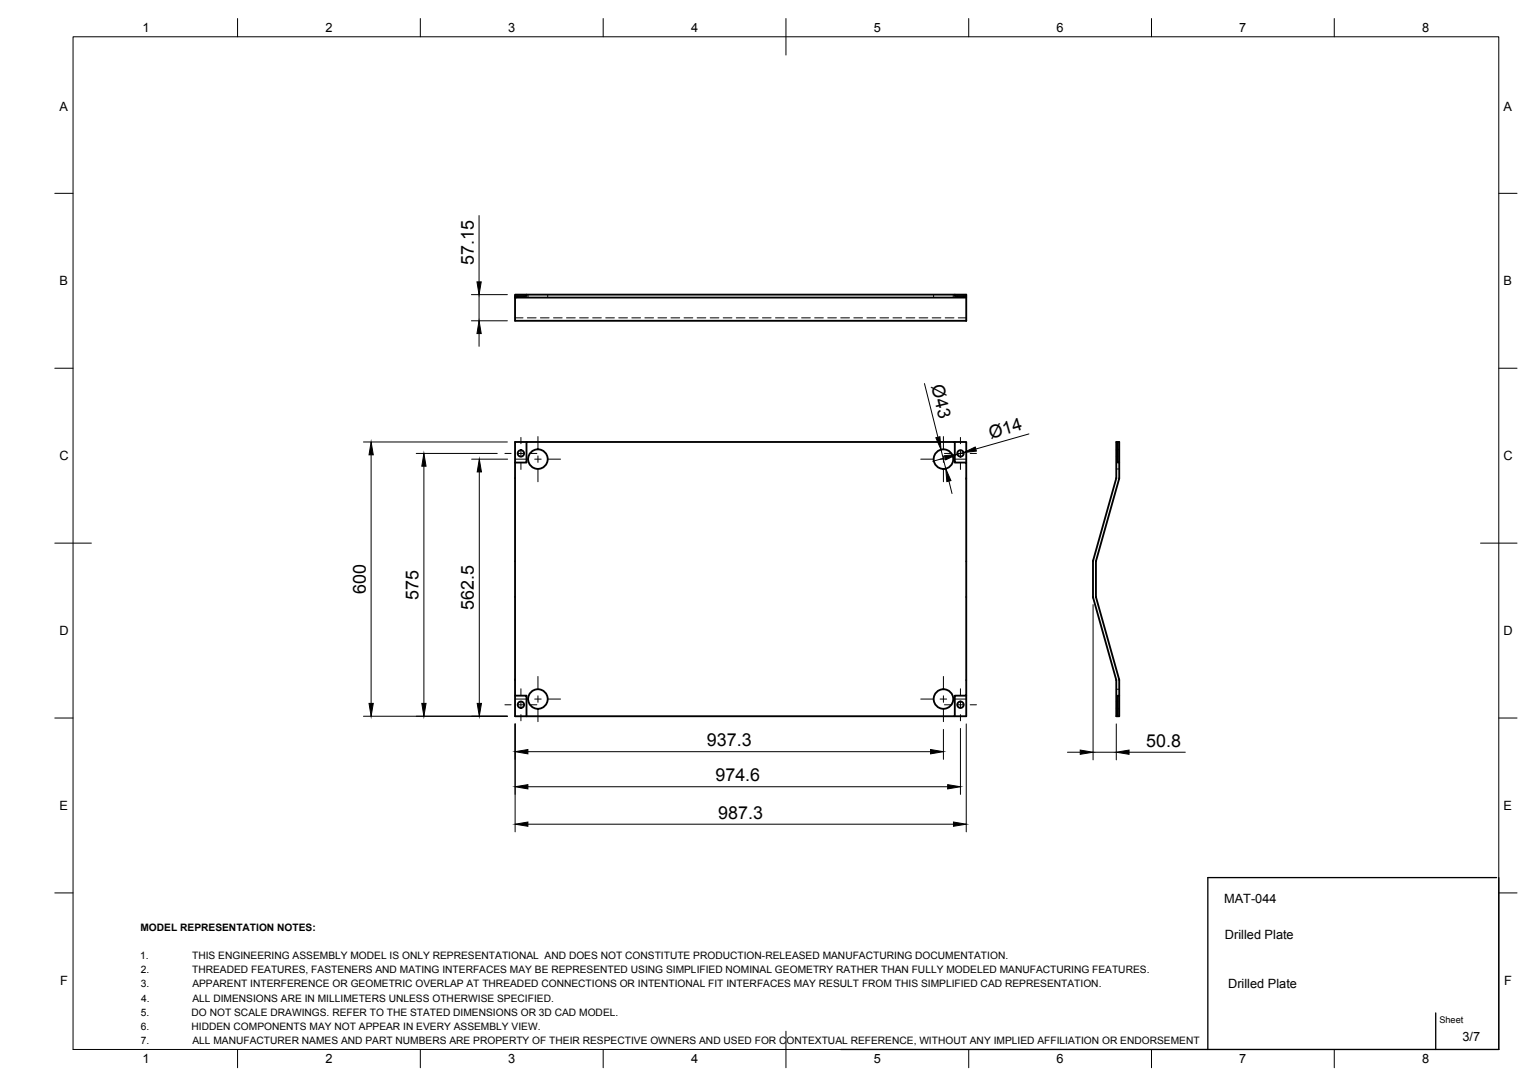
ISO-10303-21;
HEADER;
/* Generated by software containing ST-Developer
 * from STEP Tools, Inc. (www.steptools.com) 
 */

FILE_DESCRIPTION(
/* description */ ('STEP AP214'),
/* implementation_level */ '2;1');

FILE_NAME(
/* name */ 'Drilled Plate.step',
/* time_stamp */ '2026-11-14T22:20:24-08:00',
/* author */ (''),
/* organization */ (''),
/* preprocessor_version */ 'ST-DEVELOPER v20.2',
/* originating_system */ 'Autodesk Translation Framework v15.17.0.0',
/* authorisation */ '');

FILE_SCHEMA (('AUTOMOTIVE_DESIGN { 1 0 10303 214 3 1 1 }'));
ENDSEC;

DATA;
#10=MECHANICAL_DESIGN_GEOMETRIC_PRESENTATION_REPRESENTATION('',(#82),#2794);
#72=SHAPE_REPRESENTATION_RELATIONSHIP('SRR','None',#2827,#77);
#77=ADVANCED_BREP_SHAPE_REPRESENTATION('',(#87),#2789);
#82=STYLED_ITEM('',(#2861),#87);
#87=MANIFOLD_SOLID_BREP('Body1',#1641);
#92=FACE_BOUND('',#286,.T.);
#93=FACE_BOUND('',#287,.T.);
#94=FACE_BOUND('',#288,.T.);
#95=FACE_BOUND('',#289,.T.);
#96=FACE_BOUND('',#291,.T.);
#97=FACE_BOUND('',#292,.T.);
#98=FACE_BOUND('',#293,.T.);
#99=FACE_BOUND('',#294,.T.);
#100=FACE_BOUND('',#296,.T.);
#101=FACE_BOUND('',#297,.T.);
#102=FACE_BOUND('',#299,.T.);
#103=FACE_BOUND('',#300,.T.);
#104=FACE_BOUND('',#338,.T.);
#105=FACE_BOUND('',#342,.T.);
#106=FACE_BOUND('',#346,.T.);
#107=FACE_BOUND('',#350,.T.);
#116=PLANE('',#1728);
#117=PLANE('',#1729);
#118=PLANE('',#1730);
#119=PLANE('',#1731);
#120=PLANE('',#1732);
#121=PLANE('',#1733);
#122=PLANE('',#1734);
#123=PLANE('',#1735);
#124=PLANE('',#1736);
#125=PLANE('',#1739);
#126=PLANE('',#1740);
#127=PLANE('',#1743);
#128=PLANE('',#1746);
#129=PLANE('',#1747);
#130=PLANE('',#1750);
#131=PLANE('',#1751);
#132=PLANE('',#1754);
#133=PLANE('',#1755);
#134=PLANE('',#1758);
#135=PLANE('',#1759);
#136=PLANE('',#1762);
#137=PLANE('',#1765);
#138=PLANE('',#1767);
#139=PLANE('',#1769);
#140=PLANE('',#1771);
#141=PLANE('',#1774);
#142=PLANE('',#1776);
#143=PLANE('',#1778);
#144=PLANE('',#1780);
#145=PLANE('',#1781);
#146=PLANE('',#1782);
#147=PLANE('',#1783);
#148=PLANE('',#1784);
#149=PLANE('',#1785);
#150=PLANE('',#1786);
#151=PLANE('',#1787);
#152=PLANE('',#1788);
#153=PLANE('',#1789);
#154=PLANE('',#1790);
#155=PLANE('',#1791);
#156=PLANE('',#1792);
#157=PLANE('',#1793);
#186=FACE_OUTER_BOUND('',#277,.T.);
#187=FACE_OUTER_BOUND('',#278,.T.);
#188=FACE_OUTER_BOUND('',#279,.T.);
#189=FACE_OUTER_BOUND('',#280,.T.);
#190=FACE_OUTER_BOUND('',#281,.T.);
#191=FACE_OUTER_BOUND('',#282,.T.);
#192=FACE_OUTER_BOUND('',#283,.T.);
#193=FACE_OUTER_BOUND('',#284,.T.);
#194=FACE_OUTER_BOUND('',#285,.T.);
#195=FACE_OUTER_BOUND('',#290,.T.);
#196=FACE_OUTER_BOUND('',#295,.T.);
#197=FACE_OUTER_BOUND('',#298,.T.);
#198=FACE_OUTER_BOUND('',#301,.T.);
#199=FACE_OUTER_BOUND('',#302,.T.);
#200=FACE_OUTER_BOUND('',#303,.T.);
#201=FACE_OUTER_BOUND('',#304,.T.);
#202=FACE_OUTER_BOUND('',#305,.T.);
#203=FACE_OUTER_BOUND('',#306,.T.);
#204=FACE_OUTER_BOUND('',#307,.T.);
#205=FACE_OUTER_BOUND('',#308,.T.);
#206=FACE_OUTER_BOUND('',#309,.T.);
#207=FACE_OUTER_BOUND('',#310,.T.);
#208=FACE_OUTER_BOUND('',#311,.T.);
#209=FACE_OUTER_BOUND('',#312,.T.);
#210=FACE_OUTER_BOUND('',#313,.T.);
#211=FACE_OUTER_BOUND('',#314,.T.);
#212=FACE_OUTER_BOUND('',#315,.T.);
#213=FACE_OUTER_BOUND('',#316,.T.);
#214=FACE_OUTER_BOUND('',#317,.T.);
#215=FACE_OUTER_BOUND('',#318,.T.);
#216=FACE_OUTER_BOUND('',#319,.T.);
#217=FACE_OUTER_BOUND('',#320,.T.);
#218=FACE_OUTER_BOUND('',#321,.T.);
#219=FACE_OUTER_BOUND('',#322,.T.);
#220=FACE_OUTER_BOUND('',#323,.T.);
#221=FACE_OUTER_BOUND('',#324,.T.);
#222=FACE_OUTER_BOUND('',#325,.T.);
#223=FACE_OUTER_BOUND('',#326,.T.);
#224=FACE_OUTER_BOUND('',#327,.T.);
#225=FACE_OUTER_BOUND('',#328,.T.);
#226=FACE_OUTER_BOUND('',#329,.T.);
#227=FACE_OUTER_BOUND('',#330,.T.);
#228=FACE_OUTER_BOUND('',#331,.T.);
#229=FACE_OUTER_BOUND('',#332,.T.);
#230=FACE_OUTER_BOUND('',#333,.T.);
#231=FACE_OUTER_BOUND('',#334,.T.);
#232=FACE_OUTER_BOUND('',#335,.T.);
#233=FACE_OUTER_BOUND('',#336,.T.);
#234=FACE_OUTER_BOUND('',#337,.T.);
#235=FACE_OUTER_BOUND('',#339,.T.);
#236=FACE_OUTER_BOUND('',#340,.T.);
#237=FACE_OUTER_BOUND('',#341,.T.);
#238=FACE_OUTER_BOUND('',#343,.T.);
#239=FACE_OUTER_BOUND('',#344,.T.);
#240=FACE_OUTER_BOUND('',#345,.T.);
#241=FACE_OUTER_BOUND('',#347,.T.);
#242=FACE_OUTER_BOUND('',#348,.T.);
#243=FACE_OUTER_BOUND('',#349,.T.);
#277=EDGE_LOOP('',(#1110,#1111,#1112,#1113));
#278=EDGE_LOOP('',(#1114,#1115,#1116,#1117));
#279=EDGE_LOOP('',(#1118,#1119,#1120,#1121));
#280=EDGE_LOOP('',(#1122,#1123,#1124,#1125));
#281=EDGE_LOOP('',(#1126,#1127,#1128,#1129));
#282=EDGE_LOOP('',(#1130,#1131,#1132,#1133));
#283=EDGE_LOOP('',(#1134,#1135,#1136,#1137));
#284=EDGE_LOOP('',(#1138,#1139,#1140,#1141));
#285=EDGE_LOOP('',(#1142,#1143,#1144,#1145));
#286=EDGE_LOOP('',(#1146));
#287=EDGE_LOOP('',(#1147));
#288=EDGE_LOOP('',(#1148));
#289=EDGE_LOOP('',(#1149));
#290=EDGE_LOOP('',(#1150,#1151,#1152,#1153));
#291=EDGE_LOOP('',(#1154));
#292=EDGE_LOOP('',(#1155));
#293=EDGE_LOOP('',(#1156));
#294=EDGE_LOOP('',(#1157));
#295=EDGE_LOOP('',(#1158,#1159,#1160,#1161,#1162,#1163,#1164,#1165));
#296=EDGE_LOOP('',(#1166));
#297=EDGE_LOOP('',(#1167));
#298=EDGE_LOOP('',(#1168,#1169,#1170,#1171,#1172,#1173,#1174,#1175));
#299=EDGE_LOOP('',(#1176));
#300=EDGE_LOOP('',(#1177));
#301=EDGE_LOOP('',(#1178,#1179,#1180,#1181,#1182,#1183));
#302=EDGE_LOOP('',(#1184,#1185,#1186,#1187,#1188,#1189));
#303=EDGE_LOOP('',(#1190,#1191,#1192,#1193,#1194,#1195,#1196,#1197));
#304=EDGE_LOOP('',(#1198,#1199,#1200,#1201,#1202,#1203,#1204,#1205));
#305=EDGE_LOOP('',(#1206,#1207,#1208,#1209));
#306=EDGE_LOOP('',(#1210,#1211,#1212,#1213));
#307=EDGE_LOOP('',(#1214,#1215,#1216,#1217));
#308=EDGE_LOOP('',(#1218,#1219,#1220,#1221));
#309=EDGE_LOOP('',(#1222,#1223,#1224,#1225));
#310=EDGE_LOOP('',(#1226,#1227,#1228,#1229));
#311=EDGE_LOOP('',(#1230,#1231,#1232,#1233));
#312=EDGE_LOOP('',(#1234,#1235,#1236,#1237));
#313=EDGE_LOOP('',(#1238,#1239,#1240,#1241));
#314=EDGE_LOOP('',(#1242,#1243,#1244,#1245));
#315=EDGE_LOOP('',(#1246,#1247,#1248,#1249));
#316=EDGE_LOOP('',(#1250,#1251,#1252,#1253));
#317=EDGE_LOOP('',(#1254,#1255,#1256,#1257));
#318=EDGE_LOOP('',(#1258,#1259,#1260,#1261));
#319=EDGE_LOOP('',(#1262,#1263,#1264,#1265));
#320=EDGE_LOOP('',(#1266,#1267,#1268,#1269));
#321=EDGE_LOOP('',(#1270,#1271,#1272,#1273));
#322=EDGE_LOOP('',(#1274,#1275,#1276,#1277));
#323=EDGE_LOOP('',(#1278,#1279,#1280,#1281));
#324=EDGE_LOOP('',(#1282,#1283,#1284,#1285));
#325=EDGE_LOOP('',(#1286,#1287,#1288,#1289));
#326=EDGE_LOOP('',(#1290,#1291,#1292,#1293));
#327=EDGE_LOOP('',(#1294,#1295,#1296,#1297));
#328=EDGE_LOOP('',(#1298,#1299,#1300,#1301));
#329=EDGE_LOOP('',(#1302,#1303,#1304,#1305));
#330=EDGE_LOOP('',(#1306,#1307,#1308,#1309));
#331=EDGE_LOOP('',(#1310,#1311,#1312,#1313));
#332=EDGE_LOOP('',(#1314,#1315,#1316,#1317));
#333=EDGE_LOOP('',(#1318,#1319,#1320,#1321,#1322,#1323));
#334=EDGE_LOOP('',(#1324,#1325,#1326,#1327,#1328,#1329));
#335=EDGE_LOOP('',(#1330,#1331,#1332,#1333));
#336=EDGE_LOOP('',(#1334,#1335,#1336,#1337));
#337=EDGE_LOOP('',(#1338,#1339,#1340,#1341));
#338=EDGE_LOOP('',(#1342));
#339=EDGE_LOOP('',(#1343,#1344,#1345,#1346));
#340=EDGE_LOOP('',(#1347,#1348,#1349,#1350));
#341=EDGE_LOOP('',(#1351,#1352,#1353,#1354));
#342=EDGE_LOOP('',(#1355));
#343=EDGE_LOOP('',(#1356,#1357,#1358,#1359));
#344=EDGE_LOOP('',(#1360,#1361,#1362,#1363));
#345=EDGE_LOOP('',(#1364,#1365,#1366,#1367));
#346=EDGE_LOOP('',(#1368));
#347=EDGE_LOOP('',(#1369,#1370,#1371,#1372));
#348=EDGE_LOOP('',(#1373,#1374,#1375,#1376));
#349=EDGE_LOOP('',(#1377,#1378,#1379,#1380));
#350=EDGE_LOOP('',(#1381));
#392=LINE('',#2336,#561);
#393=LINE('',#2342,#562);
#394=LINE('',#2348,#563);
#395=LINE('',#2354,#564);
#396=LINE('',#2360,#565);
#397=LINE('',#2366,#566);
#398=LINE('',#2372,#567);
#399=LINE('',#2378,#568);
#400=LINE('',#2383,#569);
#401=LINE('',#2385,#570);
#402=LINE('',#2387,#571);
#403=LINE('',#2388,#572);
#404=LINE('',#2392,#573);
#405=LINE('',#2394,#574);
#406=LINE('',#2396,#575);
#407=LINE('',#2397,#576);
#408=LINE('',#2401,#577);
#409=LINE('',#2403,#578);
#410=LINE('',#2405,#579);
#411=LINE('',#2407,#580);
#412=LINE('',#2409,#581);
#413=LINE('',#2411,#582);
#414=LINE('',#2413,#583);
#415=LINE('',#2414,#584);
#416=LINE('',#2418,#585);
#417=LINE('',#2420,#586);
#418=LINE('',#2422,#587);
#419=LINE('',#2424,#588);
#420=LINE('',#2426,#589);
#421=LINE('',#2428,#590);
#422=LINE('',#2430,#591);
#423=LINE('',#2431,#592);
#424=LINE('',#2435,#593);
#425=LINE('',#2436,#594);
#426=LINE('',#2437,#595);
#427=LINE('',#2438,#596);
#428=LINE('',#2442,#597);
#429=LINE('',#2443,#598);
#430=LINE('',#2444,#599);
#431=LINE('',#2445,#600);
#432=LINE('',#2448,#601);
#433=LINE('',#2449,#602);
#434=LINE('',#2451,#603);
#435=LINE('',#2453,#604);
#436=LINE('',#2454,#605);
#437=LINE('',#2458,#606);
#438=LINE('',#2459,#607);
#439=LINE('',#2461,#608);
#440=LINE('',#2462,#609);
#441=LINE('',#2463,#610);
#442=LINE('',#2467,#611);
#443=LINE('',#2469,#612);
#444=LINE('',#2473,#613);
#445=LINE('',#2475,#614);
#446=LINE('',#2476,#615);
#447=LINE('',#2481,#616);
#448=LINE('',#2486,#617);
#449=LINE('',#2491,#618);
#450=LINE('',#2493,#619);
#451=LINE('',#2494,#620);
#452=LINE('',#2498,#621);
#453=LINE('',#2502,#622);
#454=LINE('',#2505,#623);
#455=LINE('',#2506,#624);
#456=LINE('',#2510,#625);
#457=LINE('',#2515,#626);
#458=LINE('',#2517,#627);
#459=LINE('',#2518,#628);
#460=LINE('',#2522,#629);
#461=LINE('',#2526,#630);
#462=LINE('',#2529,#631);
#463=LINE('',#2530,#632);
#464=LINE('',#2537,#633);
#465=LINE('',#2539,#634);
#466=LINE('',#2542,#635);
#467=LINE('',#2543,#636);
#468=LINE('',#2545,#637);
#469=LINE('',#2547,#638);
#470=LINE('',#2549,#639);
#471=LINE('',#2551,#640);
#472=LINE('',#2553,#641);
#473=LINE('',#2555,#642);
#474=LINE('',#2558,#643);
#475=LINE('',#2560,#644);
#476=LINE('',#2562,#645);
#477=LINE('',#2564,#646);
#478=LINE('',#2566,#647);
#479=LINE('',#2568,#648);
#480=LINE('',#2572,#649);
#481=LINE('',#2573,#650);
#482=LINE('',#2576,#651);
#483=LINE('',#2577,#652);
#484=LINE('',#2580,#653);
#485=LINE('',#2581,#654);
#486=LINE('',#2583,#655);
#487=LINE('',#2587,#656);
#488=LINE('',#2588,#657);
#489=LINE('',#2590,#658);
#490=LINE('',#2594,#659);
#491=LINE('',#2595,#660);
#492=LINE('',#2597,#661);
#493=LINE('',#2601,#662);
#494=LINE('',#2602,#663);
#495=LINE('',#2604,#664);
#561=VECTOR('',#1863,6.99999999999993);
#562=VECTOR('',#1870,7.00000000000001);
#563=VECTOR('',#1877,6.99999999999996);
#564=VECTOR('',#1884,6.9999999999999);
#565=VECTOR('',#1891,21.5);
#566=VECTOR('',#1898,21.5);
#567=VECTOR('',#1905,21.5);
#568=VECTOR('',#1912,21.5);
#569=VECTOR('',#1917,1000.);
#570=VECTOR('',#1918,1000.);
#571=VECTOR('',#1919,1000.);
#572=VECTOR('',#1920,1000.);
#573=VECTOR('',#1923,1000.);
#574=VECTOR('',#1924,1000.);
#575=VECTOR('',#1925,1000.);
#576=VECTOR('',#1926,1000.);
#577=VECTOR('',#1929,1000.);
#578=VECTOR('',#1930,1000.);
#579=VECTOR('',#1931,1000.);
#580=VECTOR('',#1932,1000.);
#581=VECTOR('',#1933,1000.);
#582=VECTOR('',#1934,1000.);
#583=VECTOR('',#1935,1000.);
#584=VECTOR('',#1936,1000.);
#585=VECTOR('',#1939,1000.);
#586=VECTOR('',#1940,1000.);
#587=VECTOR('',#1941,1000.);
#588=VECTOR('',#1942,1000.);
#589=VECTOR('',#1943,1000.);
#590=VECTOR('',#1944,1000.);
#591=VECTOR('',#1945,1000.);
#592=VECTOR('',#1946,1000.);
#593=VECTOR('',#1949,1000.);
#594=VECTOR('',#1950,1000.);
#595=VECTOR('',#1951,1000.);
#596=VECTOR('',#1952,1000.);
#597=VECTOR('',#1955,1000.);
#598=VECTOR('',#1956,1000.);
#599=VECTOR('',#1957,1000.);
#600=VECTOR('',#1958,1000.);
#601=VECTOR('',#1961,1000.);
#602=VECTOR('',#1962,1000.);
#603=VECTOR('',#1963,1000.);
#604=VECTOR('',#1964,1000.);
#605=VECTOR('',#1965,1000.);
#606=VECTOR('',#1968,1000.);
#607=VECTOR('',#1969,1000.);
#608=VECTOR('',#1970,1000.);
#609=VECTOR('',#1971,1000.);
#610=VECTOR('',#1972,1000.);
#611=VECTOR('',#1975,1000.);
#612=VECTOR('',#1978,1000.);
#613=VECTOR('',#1983,1000.);
#614=VECTOR('',#1984,1000.);
#615=VECTOR('',#1985,1000.);
#616=VECTOR('',#1990,1000.);
#617=VECTOR('',#1995,1000.);
#618=VECTOR('',#2002,1000.);
#619=VECTOR('',#2003,1000.);
#620=VECTOR('',#2004,1000.);
#621=VECTOR('',#2007,1000.);
#622=VECTOR('',#2010,1000.);
#623=VECTOR('',#2015,1000.);
#624=VECTOR('',#2016,1000.);
#625=VECTOR('',#2019,1000.);
#626=VECTOR('',#2026,1000.);
#627=VECTOR('',#2027,1000.);
#628=VECTOR('',#2028,1000.);
#629=VECTOR('',#2031,1000.);
#630=VECTOR('',#2034,1000.);
#631=VECTOR('',#2039,1000.);
#632=VECTOR('',#2040,1000.);
#633=VECTOR('',#2049,1000.);
#634=VECTOR('',#2052,1000.);
#635=VECTOR('',#2057,1000.);
#636=VECTOR('',#2058,1000.);
#637=VECTOR('',#2061,1000.);
#638=VECTOR('',#2064,1000.);
#639=VECTOR('',#2067,1000.);
#640=VECTOR('',#2070,1000.);
#641=VECTOR('',#2073,1000.);
#642=VECTOR('',#2076,1000.);
#643=VECTOR('',#2081,1000.);
#644=VECTOR('',#2084,1000.);
#645=VECTOR('',#2087,1000.);
#646=VECTOR('',#2090,1000.);
#647=VECTOR('',#2093,1000.);
#648=VECTOR('',#2096,1000.);
#649=VECTOR('',#2101,1000.);
#650=VECTOR('',#2102,1000.);
#651=VECTOR('',#2105,1000.);
#652=VECTOR('',#2106,1000.);
#653=VECTOR('',#2109,1000.);
#654=VECTOR('',#2110,1000.);
#655=VECTOR('',#2113,1000.);
#656=VECTOR('',#2118,1000.);
#657=VECTOR('',#2119,1000.);
#658=VECTOR('',#2122,1000.);
#659=VECTOR('',#2127,1000.);
#660=VECTOR('',#2128,1000.);
#661=VECTOR('',#2131,1000.);
#662=VECTOR('',#2136,1000.);
#663=VECTOR('',#2137,1000.);
#664=VECTOR('',#2140,1000.);
#730=CIRCLE('',#1705,6.99999999999992);
#731=CIRCLE('',#1706,6.99999999999992);
#732=CIRCLE('',#1708,7.00000000000001);
#733=CIRCLE('',#1709,7.00000000000001);
#734=CIRCLE('',#1711,6.99999999999996);
#735=CIRCLE('',#1712,6.99999999999996);
#736=CIRCLE('',#1714,6.9999999999999);
#737=CIRCLE('',#1715,6.9999999999999);
#738=CIRCLE('',#1717,21.5);
#739=CIRCLE('',#1718,21.5);
#740=CIRCLE('',#1720,21.5);
#741=CIRCLE('',#1721,21.5);
#742=CIRCLE('',#1723,21.5);
#743=CIRCLE('',#1724,21.5);
#744=CIRCLE('',#1726,21.5);
#745=CIRCLE('',#1727,21.5);
#746=CIRCLE('',#1737,7.35);
#747=CIRCLE('',#1738,1.);
#748=CIRCLE('',#1741,7.35);
#749=CIRCLE('',#1742,1.);
#750=CIRCLE('',#1744,1.);
#751=CIRCLE('',#1745,7.35000000000002);
#752=CIRCLE('',#1748,1.);
#753=CIRCLE('',#1749,7.35000000000002);
#754=CIRCLE('',#1752,1.);
#755=CIRCLE('',#1753,7.35000000000002);
#756=CIRCLE('',#1756,1.);
#757=CIRCLE('',#1757,7.35000000000002);
#758=CIRCLE('',#1760,7.34999999999997);
#759=CIRCLE('',#1761,1.);
#760=CIRCLE('',#1763,7.34999999999997);
#761=CIRCLE('',#1764,1.);
#771=VERTEX_POINT('',#2333);
#772=VERTEX_POINT('',#2335);
#773=VERTEX_POINT('',#2339);
#774=VERTEX_POINT('',#2341);
#775=VERTEX_POINT('',#2345);
#776=VERTEX_POINT('',#2347);
#777=VERTEX_POINT('',#2351);
#778=VERTEX_POINT('',#2353);
#779=VERTEX_POINT('',#2357);
#780=VERTEX_POINT('',#2359);
#781=VERTEX_POINT('',#2363);
#782=VERTEX_POINT('',#2365);
#783=VERTEX_POINT('',#2369);
#784=VERTEX_POINT('',#2371);
#785=VERTEX_POINT('',#2375);
#786=VERTEX_POINT('',#2377);
#787=VERTEX_POINT('',#2381);
#788=VERTEX_POINT('',#2382);
#789=VERTEX_POINT('',#2384);
#790=VERTEX_POINT('',#2386);
#791=VERTEX_POINT('',#2390);
#792=VERTEX_POINT('',#2391);
#793=VERTEX_POINT('',#2393);
#794=VERTEX_POINT('',#2395);
#795=VERTEX_POINT('',#2399);
#796=VERTEX_POINT('',#2400);
#797=VERTEX_POINT('',#2402);
#798=VERTEX_POINT('',#2404);
#799=VERTEX_POINT('',#2406);
#800=VERTEX_POINT('',#2408);
#801=VERTEX_POINT('',#2410);
#802=VERTEX_POINT('',#2412);
#803=VERTEX_POINT('',#2416);
#804=VERTEX_POINT('',#2417);
#805=VERTEX_POINT('',#2419);
#806=VERTEX_POINT('',#2421);
#807=VERTEX_POINT('',#2423);
#808=VERTEX_POINT('',#2425);
#809=VERTEX_POINT('',#2427);
#810=VERTEX_POINT('',#2429);
#811=VERTEX_POINT('',#2433);
#812=VERTEX_POINT('',#2434);
#813=VERTEX_POINT('',#2440);
#814=VERTEX_POINT('',#2441);
#815=VERTEX_POINT('',#2447);
#816=VERTEX_POINT('',#2450);
#817=VERTEX_POINT('',#2452);
#818=VERTEX_POINT('',#2456);
#819=VERTEX_POINT('',#2457);
#820=VERTEX_POINT('',#2460);
#821=VERTEX_POINT('',#2465);
#822=VERTEX_POINT('',#2466);
#823=VERTEX_POINT('',#2472);
#824=VERTEX_POINT('',#2474);
#825=VERTEX_POINT('',#2478);
#826=VERTEX_POINT('',#2480);
#827=VERTEX_POINT('',#2484);
#828=VERTEX_POINT('',#2485);
#829=VERTEX_POINT('',#2490);
#830=VERTEX_POINT('',#2492);
#831=VERTEX_POINT('',#2496);
#832=VERTEX_POINT('',#2497);
#833=VERTEX_POINT('',#2499);
#834=VERTEX_POINT('',#2501);
#835=VERTEX_POINT('',#2508);
#836=VERTEX_POINT('',#2509);
#837=VERTEX_POINT('',#2514);
#838=VERTEX_POINT('',#2516);
#839=VERTEX_POINT('',#2520);
#840=VERTEX_POINT('',#2521);
#841=VERTEX_POINT('',#2523);
#842=VERTEX_POINT('',#2525);
#843=VERTEX_POINT('',#2535);
#844=VERTEX_POINT('',#2536);
#845=VERTEX_POINT('',#2571);
#846=VERTEX_POINT('',#2575);
#847=VERTEX_POINT('',#2579);
#848=VERTEX_POINT('',#2586);
#849=VERTEX_POINT('',#2593);
#850=VERTEX_POINT('',#2600);
#900=EDGE_CURVE('',#771,#771,#730,.T.);
#901=EDGE_CURVE('',#771,#772,#392,.T.);
#902=EDGE_CURVE('',#772,#772,#731,.T.);
#903=EDGE_CURVE('',#773,#773,#732,.T.);
#904=EDGE_CURVE('',#773,#774,#393,.T.);
#905=EDGE_CURVE('',#774,#774,#733,.T.);
#906=EDGE_CURVE('',#775,#775,#734,.T.);
#907=EDGE_CURVE('',#775,#776,#394,.T.);
#908=EDGE_CURVE('',#776,#776,#735,.T.);
#909=EDGE_CURVE('',#777,#777,#736,.T.);
#910=EDGE_CURVE('',#777,#778,#395,.T.);
#911=EDGE_CURVE('',#778,#778,#737,.T.);
#912=EDGE_CURVE('',#779,#779,#738,.T.);
#913=EDGE_CURVE('',#779,#780,#396,.T.);
#914=EDGE_CURVE('',#780,#780,#739,.T.);
#915=EDGE_CURVE('',#781,#781,#740,.T.);
#916=EDGE_CURVE('',#781,#782,#397,.T.);
#917=EDGE_CURVE('',#782,#782,#741,.T.);
#918=EDGE_CURVE('',#783,#783,#742,.T.);
#919=EDGE_CURVE('',#783,#784,#398,.T.);
#920=EDGE_CURVE('',#784,#784,#743,.T.);
#921=EDGE_CURVE('',#785,#785,#744,.T.);
#922=EDGE_CURVE('',#785,#786,#399,.T.);
#923=EDGE_CURVE('',#786,#786,#745,.T.);
#924=EDGE_CURVE('',#787,#788,#400,.T.);
#925=EDGE_CURVE('',#789,#788,#401,.T.);
#926=EDGE_CURVE('',#790,#789,#402,.T.);
#927=EDGE_CURVE('',#790,#787,#403,.T.);
#928=EDGE_CURVE('',#791,#792,#404,.T.);
#929=EDGE_CURVE('',#793,#792,#405,.T.);
#930=EDGE_CURVE('',#794,#793,#406,.T.);
#931=EDGE_CURVE('',#794,#791,#407,.T.);
#932=EDGE_CURVE('',#795,#796,#408,.T.);
#933=EDGE_CURVE('',#796,#797,#409,.T.);
#934=EDGE_CURVE('',#798,#797,#410,.T.);
#935=EDGE_CURVE('',#798,#799,#411,.T.);
#936=EDGE_CURVE('',#799,#800,#412,.T.);
#937=EDGE_CURVE('',#801,#800,#413,.T.);
#938=EDGE_CURVE('',#802,#801,#414,.T.);
#939=EDGE_CURVE('',#795,#802,#415,.T.);
#940=EDGE_CURVE('',#803,#804,#416,.T.);
#941=EDGE_CURVE('',#803,#805,#417,.T.);
#942=EDGE_CURVE('',#806,#805,#418,.T.);
#943=EDGE_CURVE('',#806,#807,#419,.T.);
#944=EDGE_CURVE('',#807,#808,#420,.T.);
#945=EDGE_CURVE('',#809,#808,#421,.T.);
#946=EDGE_CURVE('',#809,#810,#422,.T.);
#947=EDGE_CURVE('',#804,#810,#423,.T.);
#948=EDGE_CURVE('',#811,#812,#424,.T.);
#949=EDGE_CURVE('',#811,#809,#425,.T.);
#950=EDGE_CURVE('',#808,#792,#426,.T.);
#951=EDGE_CURVE('',#791,#812,#427,.T.);
#952=EDGE_CURVE('',#813,#814,#428,.T.);
#953=EDGE_CURVE('',#814,#796,#429,.T.);
#954=EDGE_CURVE('',#795,#790,#430,.T.);
#955=EDGE_CURVE('',#813,#789,#431,.T.);
#956=EDGE_CURVE('',#815,#798,#432,.T.);
#957=EDGE_CURVE('',#813,#815,#433,.T.);
#958=EDGE_CURVE('',#816,#788,#434,.T.);
#959=EDGE_CURVE('',#816,#817,#435,.T.);
#960=EDGE_CURVE('',#817,#799,#436,.T.);
#961=EDGE_CURVE('',#818,#819,#437,.T.);
#962=EDGE_CURVE('',#818,#803,#438,.T.);
#963=EDGE_CURVE('',#820,#804,#439,.T.);
#964=EDGE_CURVE('',#812,#820,#440,.T.);
#965=EDGE_CURVE('',#794,#819,#441,.T.);
#966=EDGE_CURVE('',#821,#822,#442,.T.);
#967=EDGE_CURVE('',#807,#821,#746,.T.);
#968=EDGE_CURVE('',#793,#807,#443,.T.);
#969=EDGE_CURVE('',#793,#822,#747,.T.);
#970=EDGE_CURVE('',#821,#823,#444,.T.);
#971=EDGE_CURVE('',#822,#824,#445,.T.);
#972=EDGE_CURVE('',#824,#823,#446,.T.);
#973=EDGE_CURVE('',#808,#825,#748,.T.);
#974=EDGE_CURVE('',#826,#825,#447,.T.);
#975=EDGE_CURVE('',#792,#826,#749,.T.);
#976=EDGE_CURVE('',#827,#828,#448,.T.);
#977=EDGE_CURVE('',#823,#827,#750,.T.);
#978=EDGE_CURVE('',#824,#828,#751,.T.);
#979=EDGE_CURVE('',#827,#829,#449,.T.);
#980=EDGE_CURVE('',#828,#830,#450,.T.);
#981=EDGE_CURVE('',#830,#829,#451,.T.);
#982=EDGE_CURVE('',#831,#832,#452,.T.);
#983=EDGE_CURVE('',#831,#833,#752,.T.);
#984=EDGE_CURVE('',#834,#833,#453,.T.);
#985=EDGE_CURVE('',#832,#834,#753,.T.);
#986=EDGE_CURVE('',#825,#831,#454,.T.);
#987=EDGE_CURVE('',#826,#832,#455,.T.);
#988=EDGE_CURVE('',#835,#836,#456,.T.);
#989=EDGE_CURVE('',#829,#835,#754,.T.);
#990=EDGE_CURVE('',#830,#836,#755,.T.);
#991=EDGE_CURVE('',#835,#837,#457,.T.);
#992=EDGE_CURVE('',#836,#838,#458,.T.);
#993=EDGE_CURVE('',#838,#837,#459,.T.);
#994=EDGE_CURVE('',#839,#840,#460,.T.);
#995=EDGE_CURVE('',#839,#841,#756,.T.);
#996=EDGE_CURVE('',#842,#841,#461,.T.);
#997=EDGE_CURVE('',#840,#842,#757,.T.);
#998=EDGE_CURVE('',#833,#839,#462,.T.);
#999=EDGE_CURVE('',#834,#840,#463,.T.);
#1000=EDGE_CURVE('',#837,#795,#758,.T.);
#1001=EDGE_CURVE('',#838,#790,#759,.T.);
#1002=EDGE_CURVE('',#843,#844,#464,.T.);
#1003=EDGE_CURVE('',#843,#802,#760,.T.);
#1004=EDGE_CURVE('',#787,#802,#465,.T.);
#1005=EDGE_CURVE('',#844,#787,#761,.T.);
#1006=EDGE_CURVE('',#841,#843,#466,.T.);
#1007=EDGE_CURVE('',#842,#844,#467,.T.);
#1008=EDGE_CURVE('',#837,#843,#468,.T.);
#1009=EDGE_CURVE('',#835,#841,#469,.T.);
#1010=EDGE_CURVE('',#829,#839,#470,.T.);
#1011=EDGE_CURVE('',#827,#833,#471,.T.);
#1012=EDGE_CURVE('',#823,#831,#472,.T.);
#1013=EDGE_CURVE('',#821,#825,#473,.T.);
#1014=EDGE_CURVE('',#822,#826,#474,.T.);
#1015=EDGE_CURVE('',#824,#832,#475,.T.);
#1016=EDGE_CURVE('',#828,#834,#476,.T.);
#1017=EDGE_CURVE('',#830,#840,#477,.T.);
#1018=EDGE_CURVE('',#836,#842,#478,.T.);
#1019=EDGE_CURVE('',#838,#844,#479,.T.);
#1020=EDGE_CURVE('',#845,#806,#480,.T.);
#1021=EDGE_CURVE('',#819,#845,#481,.T.);
#1022=EDGE_CURVE('',#846,#801,#482,.T.);
#1023=EDGE_CURVE('',#816,#846,#483,.T.);
#1024=EDGE_CURVE('',#817,#847,#484,.T.);
#1025=EDGE_CURVE('',#847,#800,#485,.T.);
#1026=EDGE_CURVE('',#846,#847,#486,.T.);
#1027=EDGE_CURVE('',#818,#848,#487,.T.);
#1028=EDGE_CURVE('',#848,#805,#488,.T.);
#1029=EDGE_CURVE('',#845,#848,#489,.T.);
#1030=EDGE_CURVE('',#811,#849,#490,.T.);
#1031=EDGE_CURVE('',#849,#810,#491,.T.);
#1032=EDGE_CURVE('',#820,#849,#492,.T.);
#1033=EDGE_CURVE('',#814,#850,#493,.T.);
#1034=EDGE_CURVE('',#850,#797,#494,.T.);
#1035=EDGE_CURVE('',#815,#850,#495,.T.);
#1110=ORIENTED_EDGE('',*,*,#900,.F.);
#1111=ORIENTED_EDGE('',*,*,#901,.T.);
#1112=ORIENTED_EDGE('',*,*,#902,.T.);
#1113=ORIENTED_EDGE('',*,*,#901,.F.);
#1114=ORIENTED_EDGE('',*,*,#903,.F.);
#1115=ORIENTED_EDGE('',*,*,#904,.T.);
#1116=ORIENTED_EDGE('',*,*,#905,.T.);
#1117=ORIENTED_EDGE('',*,*,#904,.F.);
#1118=ORIENTED_EDGE('',*,*,#906,.T.);
#1119=ORIENTED_EDGE('',*,*,#907,.T.);
#1120=ORIENTED_EDGE('',*,*,#908,.F.);
#1121=ORIENTED_EDGE('',*,*,#907,.F.);
#1122=ORIENTED_EDGE('',*,*,#909,.T.);
#1123=ORIENTED_EDGE('',*,*,#910,.T.);
#1124=ORIENTED_EDGE('',*,*,#911,.F.);
#1125=ORIENTED_EDGE('',*,*,#910,.F.);
#1126=ORIENTED_EDGE('',*,*,#912,.T.);
#1127=ORIENTED_EDGE('',*,*,#913,.T.);
#1128=ORIENTED_EDGE('',*,*,#914,.F.);
#1129=ORIENTED_EDGE('',*,*,#913,.F.);
#1130=ORIENTED_EDGE('',*,*,#915,.F.);
#1131=ORIENTED_EDGE('',*,*,#916,.T.);
#1132=ORIENTED_EDGE('',*,*,#917,.T.);
#1133=ORIENTED_EDGE('',*,*,#916,.F.);
#1134=ORIENTED_EDGE('',*,*,#918,.T.);
#1135=ORIENTED_EDGE('',*,*,#919,.T.);
#1136=ORIENTED_EDGE('',*,*,#920,.F.);
#1137=ORIENTED_EDGE('',*,*,#919,.F.);
#1138=ORIENTED_EDGE('',*,*,#921,.F.);
#1139=ORIENTED_EDGE('',*,*,#922,.T.);
#1140=ORIENTED_EDGE('',*,*,#923,.T.);
#1141=ORIENTED_EDGE('',*,*,#922,.F.);
#1142=ORIENTED_EDGE('',*,*,#924,.T.);
#1143=ORIENTED_EDGE('',*,*,#925,.F.);
#1144=ORIENTED_EDGE('',*,*,#926,.F.);
#1145=ORIENTED_EDGE('',*,*,#927,.T.);
#1146=ORIENTED_EDGE('',*,*,#915,.T.);
#1147=ORIENTED_EDGE('',*,*,#902,.F.);
#1148=ORIENTED_EDGE('',*,*,#911,.T.);
#1149=ORIENTED_EDGE('',*,*,#912,.F.);
#1150=ORIENTED_EDGE('',*,*,#928,.T.);
#1151=ORIENTED_EDGE('',*,*,#929,.F.);
#1152=ORIENTED_EDGE('',*,*,#930,.F.);
#1153=ORIENTED_EDGE('',*,*,#931,.T.);
#1154=ORIENTED_EDGE('',*,*,#921,.T.);
#1155=ORIENTED_EDGE('',*,*,#905,.F.);
#1156=ORIENTED_EDGE('',*,*,#908,.T.);
#1157=ORIENTED_EDGE('',*,*,#918,.F.);
#1158=ORIENTED_EDGE('',*,*,#932,.T.);
#1159=ORIENTED_EDGE('',*,*,#933,.T.);
#1160=ORIENTED_EDGE('',*,*,#934,.F.);
#1161=ORIENTED_EDGE('',*,*,#935,.T.);
#1162=ORIENTED_EDGE('',*,*,#936,.T.);
#1163=ORIENTED_EDGE('',*,*,#937,.F.);
#1164=ORIENTED_EDGE('',*,*,#938,.F.);
#1165=ORIENTED_EDGE('',*,*,#939,.F.);
#1166=ORIENTED_EDGE('',*,*,#917,.F.);
#1167=ORIENTED_EDGE('',*,*,#914,.T.);
#1168=ORIENTED_EDGE('',*,*,#940,.F.);
#1169=ORIENTED_EDGE('',*,*,#941,.T.);
#1170=ORIENTED_EDGE('',*,*,#942,.F.);
#1171=ORIENTED_EDGE('',*,*,#943,.T.);
#1172=ORIENTED_EDGE('',*,*,#944,.T.);
#1173=ORIENTED_EDGE('',*,*,#945,.F.);
#1174=ORIENTED_EDGE('',*,*,#946,.T.);
#1175=ORIENTED_EDGE('',*,*,#947,.F.);
#1176=ORIENTED_EDGE('',*,*,#923,.F.);
#1177=ORIENTED_EDGE('',*,*,#920,.T.);
#1178=ORIENTED_EDGE('',*,*,#948,.F.);
#1179=ORIENTED_EDGE('',*,*,#949,.T.);
#1180=ORIENTED_EDGE('',*,*,#945,.T.);
#1181=ORIENTED_EDGE('',*,*,#950,.T.);
#1182=ORIENTED_EDGE('',*,*,#928,.F.);
#1183=ORIENTED_EDGE('',*,*,#951,.T.);
#1184=ORIENTED_EDGE('',*,*,#952,.T.);
#1185=ORIENTED_EDGE('',*,*,#953,.T.);
#1186=ORIENTED_EDGE('',*,*,#932,.F.);
#1187=ORIENTED_EDGE('',*,*,#954,.T.);
#1188=ORIENTED_EDGE('',*,*,#926,.T.);
#1189=ORIENTED_EDGE('',*,*,#955,.F.);
#1190=ORIENTED_EDGE('',*,*,#956,.F.);
#1191=ORIENTED_EDGE('',*,*,#957,.F.);
#1192=ORIENTED_EDGE('',*,*,#955,.T.);
#1193=ORIENTED_EDGE('',*,*,#925,.T.);
#1194=ORIENTED_EDGE('',*,*,#958,.F.);
#1195=ORIENTED_EDGE('',*,*,#959,.T.);
#1196=ORIENTED_EDGE('',*,*,#960,.T.);
#1197=ORIENTED_EDGE('',*,*,#935,.F.);
#1198=ORIENTED_EDGE('',*,*,#961,.F.);
#1199=ORIENTED_EDGE('',*,*,#962,.T.);
#1200=ORIENTED_EDGE('',*,*,#940,.T.);
#1201=ORIENTED_EDGE('',*,*,#963,.F.);
#1202=ORIENTED_EDGE('',*,*,#964,.F.);
#1203=ORIENTED_EDGE('',*,*,#951,.F.);
#1204=ORIENTED_EDGE('',*,*,#931,.F.);
#1205=ORIENTED_EDGE('',*,*,#965,.T.);
#1206=ORIENTED_EDGE('',*,*,#966,.F.);
#1207=ORIENTED_EDGE('',*,*,#967,.F.);
#1208=ORIENTED_EDGE('',*,*,#968,.F.);
#1209=ORIENTED_EDGE('',*,*,#969,.T.);
#1210=ORIENTED_EDGE('',*,*,#970,.F.);
#1211=ORIENTED_EDGE('',*,*,#966,.T.);
#1212=ORIENTED_EDGE('',*,*,#971,.T.);
#1213=ORIENTED_EDGE('',*,*,#972,.T.);
#1214=ORIENTED_EDGE('',*,*,#950,.F.);
#1215=ORIENTED_EDGE('',*,*,#973,.T.);
#1216=ORIENTED_EDGE('',*,*,#974,.F.);
#1217=ORIENTED_EDGE('',*,*,#975,.F.);
#1218=ORIENTED_EDGE('',*,*,#976,.F.);
#1219=ORIENTED_EDGE('',*,*,#977,.F.);
#1220=ORIENTED_EDGE('',*,*,#972,.F.);
#1221=ORIENTED_EDGE('',*,*,#978,.T.);
#1222=ORIENTED_EDGE('',*,*,#979,.F.);
#1223=ORIENTED_EDGE('',*,*,#976,.T.);
#1224=ORIENTED_EDGE('',*,*,#980,.T.);
#1225=ORIENTED_EDGE('',*,*,#981,.T.);
#1226=ORIENTED_EDGE('',*,*,#982,.F.);
#1227=ORIENTED_EDGE('',*,*,#983,.T.);
#1228=ORIENTED_EDGE('',*,*,#984,.F.);
#1229=ORIENTED_EDGE('',*,*,#985,.F.);
#1230=ORIENTED_EDGE('',*,*,#986,.T.);
#1231=ORIENTED_EDGE('',*,*,#982,.T.);
#1232=ORIENTED_EDGE('',*,*,#987,.F.);
#1233=ORIENTED_EDGE('',*,*,#974,.T.);
#1234=ORIENTED_EDGE('',*,*,#988,.F.);
#1235=ORIENTED_EDGE('',*,*,#989,.F.);
#1236=ORIENTED_EDGE('',*,*,#981,.F.);
#1237=ORIENTED_EDGE('',*,*,#990,.T.);
#1238=ORIENTED_EDGE('',*,*,#991,.F.);
#1239=ORIENTED_EDGE('',*,*,#988,.T.);
#1240=ORIENTED_EDGE('',*,*,#992,.T.);
#1241=ORIENTED_EDGE('',*,*,#993,.T.);
#1242=ORIENTED_EDGE('',*,*,#994,.F.);
#1243=ORIENTED_EDGE('',*,*,#995,.T.);
#1244=ORIENTED_EDGE('',*,*,#996,.F.);
#1245=ORIENTED_EDGE('',*,*,#997,.F.);
#1246=ORIENTED_EDGE('',*,*,#998,.T.);
#1247=ORIENTED_EDGE('',*,*,#994,.T.);
#1248=ORIENTED_EDGE('',*,*,#999,.F.);
#1249=ORIENTED_EDGE('',*,*,#984,.T.);
#1250=ORIENTED_EDGE('',*,*,#954,.F.);
#1251=ORIENTED_EDGE('',*,*,#1000,.F.);
#1252=ORIENTED_EDGE('',*,*,#993,.F.);
#1253=ORIENTED_EDGE('',*,*,#1001,.T.);
#1254=ORIENTED_EDGE('',*,*,#1002,.F.);
#1255=ORIENTED_EDGE('',*,*,#1003,.T.);
#1256=ORIENTED_EDGE('',*,*,#1004,.F.);
#1257=ORIENTED_EDGE('',*,*,#1005,.F.);
#1258=ORIENTED_EDGE('',*,*,#1006,.T.);
#1259=ORIENTED_EDGE('',*,*,#1002,.T.);
#1260=ORIENTED_EDGE('',*,*,#1007,.F.);
#1261=ORIENTED_EDGE('',*,*,#996,.T.);
#1262=ORIENTED_EDGE('',*,*,#1003,.F.);
#1263=ORIENTED_EDGE('',*,*,#1008,.F.);
#1264=ORIENTED_EDGE('',*,*,#1000,.T.);
#1265=ORIENTED_EDGE('',*,*,#939,.T.);
#1266=ORIENTED_EDGE('',*,*,#1006,.F.);
#1267=ORIENTED_EDGE('',*,*,#1009,.F.);
#1268=ORIENTED_EDGE('',*,*,#991,.T.);
#1269=ORIENTED_EDGE('',*,*,#1008,.T.);
#1270=ORIENTED_EDGE('',*,*,#995,.F.);
#1271=ORIENTED_EDGE('',*,*,#1010,.F.);
#1272=ORIENTED_EDGE('',*,*,#989,.T.);
#1273=ORIENTED_EDGE('',*,*,#1009,.T.);
#1274=ORIENTED_EDGE('',*,*,#998,.F.);
#1275=ORIENTED_EDGE('',*,*,#1011,.F.);
#1276=ORIENTED_EDGE('',*,*,#979,.T.);
#1277=ORIENTED_EDGE('',*,*,#1010,.T.);
#1278=ORIENTED_EDGE('',*,*,#983,.F.);
#1279=ORIENTED_EDGE('',*,*,#1012,.F.);
#1280=ORIENTED_EDGE('',*,*,#977,.T.);
#1281=ORIENTED_EDGE('',*,*,#1011,.T.);
#1282=ORIENTED_EDGE('',*,*,#986,.F.);
#1283=ORIENTED_EDGE('',*,*,#1013,.F.);
#1284=ORIENTED_EDGE('',*,*,#970,.T.);
#1285=ORIENTED_EDGE('',*,*,#1012,.T.);
#1286=ORIENTED_EDGE('',*,*,#973,.F.);
#1287=ORIENTED_EDGE('',*,*,#944,.F.);
#1288=ORIENTED_EDGE('',*,*,#967,.T.);
#1289=ORIENTED_EDGE('',*,*,#1013,.T.);
#1290=ORIENTED_EDGE('',*,*,#975,.T.);
#1291=ORIENTED_EDGE('',*,*,#1014,.F.);
#1292=ORIENTED_EDGE('',*,*,#969,.F.);
#1293=ORIENTED_EDGE('',*,*,#929,.T.);
#1294=ORIENTED_EDGE('',*,*,#987,.T.);
#1295=ORIENTED_EDGE('',*,*,#1015,.F.);
#1296=ORIENTED_EDGE('',*,*,#971,.F.);
#1297=ORIENTED_EDGE('',*,*,#1014,.T.);
#1298=ORIENTED_EDGE('',*,*,#985,.T.);
#1299=ORIENTED_EDGE('',*,*,#1016,.F.);
#1300=ORIENTED_EDGE('',*,*,#978,.F.);
#1301=ORIENTED_EDGE('',*,*,#1015,.T.);
#1302=ORIENTED_EDGE('',*,*,#999,.T.);
#1303=ORIENTED_EDGE('',*,*,#1017,.F.);
#1304=ORIENTED_EDGE('',*,*,#980,.F.);
#1305=ORIENTED_EDGE('',*,*,#1016,.T.);
#1306=ORIENTED_EDGE('',*,*,#997,.T.);
#1307=ORIENTED_EDGE('',*,*,#1018,.F.);
#1308=ORIENTED_EDGE('',*,*,#990,.F.);
#1309=ORIENTED_EDGE('',*,*,#1017,.T.);
#1310=ORIENTED_EDGE('',*,*,#1007,.T.);
#1311=ORIENTED_EDGE('',*,*,#1019,.F.);
#1312=ORIENTED_EDGE('',*,*,#992,.F.);
#1313=ORIENTED_EDGE('',*,*,#1018,.T.);
#1314=ORIENTED_EDGE('',*,*,#1005,.T.);
#1315=ORIENTED_EDGE('',*,*,#927,.F.);
#1316=ORIENTED_EDGE('',*,*,#1001,.F.);
#1317=ORIENTED_EDGE('',*,*,#1019,.T.);
#1318=ORIENTED_EDGE('',*,*,#1020,.F.);
#1319=ORIENTED_EDGE('',*,*,#1021,.F.);
#1320=ORIENTED_EDGE('',*,*,#965,.F.);
#1321=ORIENTED_EDGE('',*,*,#930,.T.);
#1322=ORIENTED_EDGE('',*,*,#968,.T.);
#1323=ORIENTED_EDGE('',*,*,#943,.F.);
#1324=ORIENTED_EDGE('',*,*,#938,.T.);
#1325=ORIENTED_EDGE('',*,*,#1022,.F.);
#1326=ORIENTED_EDGE('',*,*,#1023,.F.);
#1327=ORIENTED_EDGE('',*,*,#958,.T.);
#1328=ORIENTED_EDGE('',*,*,#924,.F.);
#1329=ORIENTED_EDGE('',*,*,#1004,.T.);
#1330=ORIENTED_EDGE('',*,*,#936,.F.);
#1331=ORIENTED_EDGE('',*,*,#960,.F.);
#1332=ORIENTED_EDGE('',*,*,#1024,.T.);
#1333=ORIENTED_EDGE('',*,*,#1025,.T.);
#1334=ORIENTED_EDGE('',*,*,#937,.T.);
#1335=ORIENTED_EDGE('',*,*,#1025,.F.);
#1336=ORIENTED_EDGE('',*,*,#1026,.F.);
#1337=ORIENTED_EDGE('',*,*,#1022,.T.);
#1338=ORIENTED_EDGE('',*,*,#1023,.T.);
#1339=ORIENTED_EDGE('',*,*,#1026,.T.);
#1340=ORIENTED_EDGE('',*,*,#1024,.F.);
#1341=ORIENTED_EDGE('',*,*,#959,.F.);
#1342=ORIENTED_EDGE('',*,*,#900,.T.);
#1343=ORIENTED_EDGE('',*,*,#941,.F.);
#1344=ORIENTED_EDGE('',*,*,#962,.F.);
#1345=ORIENTED_EDGE('',*,*,#1027,.T.);
#1346=ORIENTED_EDGE('',*,*,#1028,.T.);
#1347=ORIENTED_EDGE('',*,*,#942,.T.);
#1348=ORIENTED_EDGE('',*,*,#1028,.F.);
#1349=ORIENTED_EDGE('',*,*,#1029,.F.);
#1350=ORIENTED_EDGE('',*,*,#1020,.T.);
#1351=ORIENTED_EDGE('',*,*,#1021,.T.);
#1352=ORIENTED_EDGE('',*,*,#1029,.T.);
#1353=ORIENTED_EDGE('',*,*,#1027,.F.);
#1354=ORIENTED_EDGE('',*,*,#961,.T.);
#1355=ORIENTED_EDGE('',*,*,#903,.T.);
#1356=ORIENTED_EDGE('',*,*,#946,.F.);
#1357=ORIENTED_EDGE('',*,*,#949,.F.);
#1358=ORIENTED_EDGE('',*,*,#1030,.T.);
#1359=ORIENTED_EDGE('',*,*,#1031,.T.);
#1360=ORIENTED_EDGE('',*,*,#947,.T.);
#1361=ORIENTED_EDGE('',*,*,#1031,.F.);
#1362=ORIENTED_EDGE('',*,*,#1032,.F.);
#1363=ORIENTED_EDGE('',*,*,#963,.T.);
#1364=ORIENTED_EDGE('',*,*,#964,.T.);
#1365=ORIENTED_EDGE('',*,*,#1032,.T.);
#1366=ORIENTED_EDGE('',*,*,#1030,.F.);
#1367=ORIENTED_EDGE('',*,*,#948,.T.);
#1368=ORIENTED_EDGE('',*,*,#906,.F.);
#1369=ORIENTED_EDGE('',*,*,#933,.F.);
#1370=ORIENTED_EDGE('',*,*,#953,.F.);
#1371=ORIENTED_EDGE('',*,*,#1033,.T.);
#1372=ORIENTED_EDGE('',*,*,#1034,.T.);
#1373=ORIENTED_EDGE('',*,*,#934,.T.);
#1374=ORIENTED_EDGE('',*,*,#1034,.F.);
#1375=ORIENTED_EDGE('',*,*,#1035,.F.);
#1376=ORIENTED_EDGE('',*,*,#956,.T.);
#1377=ORIENTED_EDGE('',*,*,#952,.F.);
#1378=ORIENTED_EDGE('',*,*,#957,.T.);
#1379=ORIENTED_EDGE('',*,*,#1035,.T.);
#1380=ORIENTED_EDGE('',*,*,#1033,.F.);
#1381=ORIENTED_EDGE('',*,*,#909,.F.);
#1530=CYLINDRICAL_SURFACE('',#1704,6.99999999999993);
#1531=CYLINDRICAL_SURFACE('',#1707,7.00000000000001);
#1532=CYLINDRICAL_SURFACE('',#1710,6.99999999999996);
#1533=CYLINDRICAL_SURFACE('',#1713,6.9999999999999);
#1534=CYLINDRICAL_SURFACE('',#1716,21.5);
#1535=CYLINDRICAL_SURFACE('',#1719,21.5);
#1536=CYLINDRICAL_SURFACE('',#1722,21.5);
#1537=CYLINDRICAL_SURFACE('',#1725,21.5);
#1538=CYLINDRICAL_SURFACE('',#1766,7.34999999999997);
#1539=CYLINDRICAL_SURFACE('',#1768,1.);
#1540=CYLINDRICAL_SURFACE('',#1770,1.);
#1541=CYLINDRICAL_SURFACE('',#1772,7.35);
#1542=CYLINDRICAL_SURFACE('',#1773,1.);
#1543=CYLINDRICAL_SURFACE('',#1775,7.35000000000002);
#1544=CYLINDRICAL_SURFACE('',#1777,7.35000000000002);
#1545=CYLINDRICAL_SURFACE('',#1779,1.);
#1550=ADVANCED_FACE('',(#186),#1530,.F.);
#1551=ADVANCED_FACE('',(#187),#1531,.F.);
#1552=ADVANCED_FACE('',(#188),#1532,.F.);
#1553=ADVANCED_FACE('',(#189),#1533,.F.);
#1554=ADVANCED_FACE('',(#190),#1534,.F.);
#1555=ADVANCED_FACE('',(#191),#1535,.F.);
#1556=ADVANCED_FACE('',(#192),#1536,.F.);
#1557=ADVANCED_FACE('',(#193),#1537,.F.);
#1558=ADVANCED_FACE('',(#194,#92,#93,#94,#95),#116,.F.);
#1559=ADVANCED_FACE('',(#195,#96,#97,#98,#99),#117,.F.);
#1560=ADVANCED_FACE('',(#196,#100,#101),#118,.T.);
#1561=ADVANCED_FACE('',(#197,#102,#103),#119,.T.);
#1562=ADVANCED_FACE('',(#198),#120,.T.);
#1563=ADVANCED_FACE('',(#199),#121,.T.);
#1564=ADVANCED_FACE('',(#200),#122,.T.);
#1565=ADVANCED_FACE('',(#201),#123,.T.);
#1566=ADVANCED_FACE('',(#202),#124,.T.);
#1567=ADVANCED_FACE('',(#203),#125,.T.);
#1568=ADVANCED_FACE('',(#204),#126,.T.);
#1569=ADVANCED_FACE('',(#205),#127,.T.);
#1570=ADVANCED_FACE('',(#206),#128,.T.);
#1571=ADVANCED_FACE('',(#207),#129,.T.);
#1572=ADVANCED_FACE('',(#208),#130,.T.);
#1573=ADVANCED_FACE('',(#209),#131,.T.);
#1574=ADVANCED_FACE('',(#210),#132,.T.);
#1575=ADVANCED_FACE('',(#211),#133,.T.);
#1576=ADVANCED_FACE('',(#212),#134,.T.);
#1577=ADVANCED_FACE('',(#213),#135,.T.);
#1578=ADVANCED_FACE('',(#214),#136,.T.);
#1579=ADVANCED_FACE('',(#215),#137,.T.);
#1580=ADVANCED_FACE('',(#216),#1538,.T.);
#1581=ADVANCED_FACE('',(#217),#138,.T.);
#1582=ADVANCED_FACE('',(#218),#1539,.F.);
#1583=ADVANCED_FACE('',(#219),#139,.T.);
#1584=ADVANCED_FACE('',(#220),#1540,.F.);
#1585=ADVANCED_FACE('',(#221),#140,.T.);
#1586=ADVANCED_FACE('',(#222),#1541,.T.);
#1587=ADVANCED_FACE('',(#223),#1542,.F.);
#1588=ADVANCED_FACE('',(#224),#141,.F.);
#1589=ADVANCED_FACE('',(#225),#1543,.T.);
#1590=ADVANCED_FACE('',(#226),#142,.F.);
#1591=ADVANCED_FACE('',(#227),#1544,.T.);
#1592=ADVANCED_FACE('',(#228),#143,.F.);
#1593=ADVANCED_FACE('',(#229),#1545,.F.);
#1594=ADVANCED_FACE('',(#230),#144,.T.);
#1595=ADVANCED_FACE('',(#231),#145,.F.);
#1596=ADVANCED_FACE('',(#232),#146,.T.);
#1597=ADVANCED_FACE('',(#233),#147,.F.);
#1598=ADVANCED_FACE('',(#234,#104),#148,.T.);
#1599=ADVANCED_FACE('',(#235),#149,.T.);
#1600=ADVANCED_FACE('',(#236),#150,.F.);
#1601=ADVANCED_FACE('',(#237,#105),#151,.T.);
#1602=ADVANCED_FACE('',(#238),#152,.T.);
#1603=ADVANCED_FACE('',(#239),#153,.F.);
#1604=ADVANCED_FACE('',(#240,#106),#154,.T.);
#1605=ADVANCED_FACE('',(#241),#155,.T.);
#1606=ADVANCED_FACE('',(#242),#156,.F.);
#1607=ADVANCED_FACE('',(#243,#107),#157,.T.);
#1641=CLOSED_SHELL('',(#1550,#1551,#1552,#1553,#1554,#1555,#1556,#1557,
#1558,#1559,#1560,#1561,#1562,#1563,#1564,#1565,#1566,#1567,#1568,#1569,
#1570,#1571,#1572,#1573,#1574,#1575,#1576,#1577,#1578,#1579,#1580,#1581,
#1582,#1583,#1584,#1585,#1586,#1587,#1588,#1589,#1590,#1591,#1592,#1593,
#1594,#1595,#1596,#1597,#1598,#1599,#1600,#1601,#1602,#1603,#1604,#1605,
#1606,#1607));
#1703=AXIS2_PLACEMENT_3D('',#2331,#1857,#1858);
#1704=AXIS2_PLACEMENT_3D('',#2332,#1859,#1860);
#1705=AXIS2_PLACEMENT_3D('',#2334,#1861,#1862);
#1706=AXIS2_PLACEMENT_3D('',#2337,#1864,#1865);
#1707=AXIS2_PLACEMENT_3D('',#2338,#1866,#1867);
#1708=AXIS2_PLACEMENT_3D('',#2340,#1868,#1869);
#1709=AXIS2_PLACEMENT_3D('',#2343,#1871,#1872);
#1710=AXIS2_PLACEMENT_3D('',#2344,#1873,#1874);
#1711=AXIS2_PLACEMENT_3D('',#2346,#1875,#1876);
#1712=AXIS2_PLACEMENT_3D('',#2349,#1878,#1879);
#1713=AXIS2_PLACEMENT_3D('',#2350,#1880,#1881);
#1714=AXIS2_PLACEMENT_3D('',#2352,#1882,#1883);
#1715=AXIS2_PLACEMENT_3D('',#2355,#1885,#1886);
#1716=AXIS2_PLACEMENT_3D('',#2356,#1887,#1888);
#1717=AXIS2_PLACEMENT_3D('',#2358,#1889,#1890);
#1718=AXIS2_PLACEMENT_3D('',#2361,#1892,#1893);
#1719=AXIS2_PLACEMENT_3D('',#2362,#1894,#1895);
#1720=AXIS2_PLACEMENT_3D('',#2364,#1896,#1897);
#1721=AXIS2_PLACEMENT_3D('',#2367,#1899,#1900);
#1722=AXIS2_PLACEMENT_3D('',#2368,#1901,#1902);
#1723=AXIS2_PLACEMENT_3D('',#2370,#1903,#1904);
#1724=AXIS2_PLACEMENT_3D('',#2373,#1906,#1907);
#1725=AXIS2_PLACEMENT_3D('',#2374,#1908,#1909);
#1726=AXIS2_PLACEMENT_3D('',#2376,#1910,#1911);
#1727=AXIS2_PLACEMENT_3D('',#2379,#1913,#1914);
#1728=AXIS2_PLACEMENT_3D('',#2380,#1915,#1916);
#1729=AXIS2_PLACEMENT_3D('',#2389,#1921,#1922);
#1730=AXIS2_PLACEMENT_3D('',#2398,#1927,#1928);
#1731=AXIS2_PLACEMENT_3D('',#2415,#1937,#1938);
#1732=AXIS2_PLACEMENT_3D('',#2432,#1947,#1948);
#1733=AXIS2_PLACEMENT_3D('',#2439,#1953,#1954);
#1734=AXIS2_PLACEMENT_3D('',#2446,#1959,#1960);
#1735=AXIS2_PLACEMENT_3D('',#2455,#1966,#1967);
#1736=AXIS2_PLACEMENT_3D('',#2464,#1973,#1974);
#1737=AXIS2_PLACEMENT_3D('',#2468,#1976,#1977);
#1738=AXIS2_PLACEMENT_3D('',#2470,#1979,#1980);
#1739=AXIS2_PLACEMENT_3D('',#2471,#1981,#1982);
#1740=AXIS2_PLACEMENT_3D('',#2477,#1986,#1987);
#1741=AXIS2_PLACEMENT_3D('',#2479,#1988,#1989);
#1742=AXIS2_PLACEMENT_3D('',#2482,#1991,#1992);
#1743=AXIS2_PLACEMENT_3D('',#2483,#1993,#1994);
#1744=AXIS2_PLACEMENT_3D('',#2487,#1996,#1997);
#1745=AXIS2_PLACEMENT_3D('',#2488,#1998,#1999);
#1746=AXIS2_PLACEMENT_3D('',#2489,#2000,#2001);
#1747=AXIS2_PLACEMENT_3D('',#2495,#2005,#2006);
#1748=AXIS2_PLACEMENT_3D('',#2500,#2008,#2009);
#1749=AXIS2_PLACEMENT_3D('',#2503,#2011,#2012);
#1750=AXIS2_PLACEMENT_3D('',#2504,#2013,#2014);
#1751=AXIS2_PLACEMENT_3D('',#2507,#2017,#2018);
#1752=AXIS2_PLACEMENT_3D('',#2511,#2020,#2021);
#1753=AXIS2_PLACEMENT_3D('',#2512,#2022,#2023);
#1754=AXIS2_PLACEMENT_3D('',#2513,#2024,#2025);
#1755=AXIS2_PLACEMENT_3D('',#2519,#2029,#2030);
#1756=AXIS2_PLACEMENT_3D('',#2524,#2032,#2033);
#1757=AXIS2_PLACEMENT_3D('',#2527,#2035,#2036);
#1758=AXIS2_PLACEMENT_3D('',#2528,#2037,#2038);
#1759=AXIS2_PLACEMENT_3D('',#2531,#2041,#2042);
#1760=AXIS2_PLACEMENT_3D('',#2532,#2043,#2044);
#1761=AXIS2_PLACEMENT_3D('',#2533,#2045,#2046);
#1762=AXIS2_PLACEMENT_3D('',#2534,#2047,#2048);
#1763=AXIS2_PLACEMENT_3D('',#2538,#2050,#2051);
#1764=AXIS2_PLACEMENT_3D('',#2540,#2053,#2054);
#1765=AXIS2_PLACEMENT_3D('',#2541,#2055,#2056);
#1766=AXIS2_PLACEMENT_3D('',#2544,#2059,#2060);
#1767=AXIS2_PLACEMENT_3D('',#2546,#2062,#2063);
#1768=AXIS2_PLACEMENT_3D('',#2548,#2065,#2066);
#1769=AXIS2_PLACEMENT_3D('',#2550,#2068,#2069);
#1770=AXIS2_PLACEMENT_3D('',#2552,#2071,#2072);
#1771=AXIS2_PLACEMENT_3D('',#2554,#2074,#2075);
#1772=AXIS2_PLACEMENT_3D('',#2556,#2077,#2078);
#1773=AXIS2_PLACEMENT_3D('',#2557,#2079,#2080);
#1774=AXIS2_PLACEMENT_3D('',#2559,#2082,#2083);
#1775=AXIS2_PLACEMENT_3D('',#2561,#2085,#2086);
#1776=AXIS2_PLACEMENT_3D('',#2563,#2088,#2089);
#1777=AXIS2_PLACEMENT_3D('',#2565,#2091,#2092);
#1778=AXIS2_PLACEMENT_3D('',#2567,#2094,#2095);
#1779=AXIS2_PLACEMENT_3D('',#2569,#2097,#2098);
#1780=AXIS2_PLACEMENT_3D('',#2570,#2099,#2100);
#1781=AXIS2_PLACEMENT_3D('',#2574,#2103,#2104);
#1782=AXIS2_PLACEMENT_3D('',#2578,#2107,#2108);
#1783=AXIS2_PLACEMENT_3D('',#2582,#2111,#2112);
#1784=AXIS2_PLACEMENT_3D('',#2584,#2114,#2115);
#1785=AXIS2_PLACEMENT_3D('',#2585,#2116,#2117);
#1786=AXIS2_PLACEMENT_3D('',#2589,#2120,#2121);
#1787=AXIS2_PLACEMENT_3D('',#2591,#2123,#2124);
#1788=AXIS2_PLACEMENT_3D('',#2592,#2125,#2126);
#1789=AXIS2_PLACEMENT_3D('',#2596,#2129,#2130);
#1790=AXIS2_PLACEMENT_3D('',#2598,#2132,#2133);
#1791=AXIS2_PLACEMENT_3D('',#2599,#2134,#2135);
#1792=AXIS2_PLACEMENT_3D('',#2603,#2138,#2139);
#1793=AXIS2_PLACEMENT_3D('',#2605,#2141,#2142);
#1857=DIRECTION('axis',(0.,0.,1.));
#1858=DIRECTION('refdir',(1.,0.,0.));
#1859=DIRECTION('center_axis',(0.,-1.,0.));
#1860=DIRECTION('ref_axis',(0.,0.,-1.));
#1861=DIRECTION('center_axis',(0.,-1.,0.));
#1862=DIRECTION('ref_axis',(0.,0.,1.));
#1863=DIRECTION('',(0.,-1.,0.));
#1864=DIRECTION('center_axis',(0.,-1.,0.));
#1865=DIRECTION('ref_axis',(0.,0.,1.));
#1866=DIRECTION('center_axis',(0.,-1.,0.));
#1867=DIRECTION('ref_axis',(0.,0.,-1.));
#1868=DIRECTION('center_axis',(0.,-1.,0.));
#1869=DIRECTION('ref_axis',(0.,0.,1.));
#1870=DIRECTION('',(0.,-1.,0.));
#1871=DIRECTION('center_axis',(0.,-1.,0.));
#1872=DIRECTION('ref_axis',(0.,0.,1.));
#1873=DIRECTION('center_axis',(0.,-1.,0.));
#1874=DIRECTION('ref_axis',(0.,0.,-1.));
#1875=DIRECTION('center_axis',(0.,1.,0.));
#1876=DIRECTION('ref_axis',(0.,0.,1.));
#1877=DIRECTION('',(0.,-1.,0.));
#1878=DIRECTION('center_axis',(0.,1.,0.));
#1879=DIRECTION('ref_axis',(0.,0.,1.));
#1880=DIRECTION('center_axis',(0.,-1.,0.));
#1881=DIRECTION('ref_axis',(0.,0.,-1.));
#1882=DIRECTION('center_axis',(0.,1.,0.));
#1883=DIRECTION('ref_axis',(0.,0.,1.));
#1884=DIRECTION('',(0.,-1.,0.));
#1885=DIRECTION('center_axis',(0.,1.,0.));
#1886=DIRECTION('ref_axis',(0.,0.,1.));
#1887=DIRECTION('center_axis',(0.,1.,0.));
#1888=DIRECTION('ref_axis',(0.,0.,1.));
#1889=DIRECTION('center_axis',(0.,-1.,0.));
#1890=DIRECTION('ref_axis',(0.,0.,1.));
#1891=DIRECTION('',(0.,1.,0.));
#1892=DIRECTION('center_axis',(0.,-1.,0.));
#1893=DIRECTION('ref_axis',(0.,0.,1.));
#1894=DIRECTION('center_axis',(0.,1.,0.));
#1895=DIRECTION('ref_axis',(0.,0.,1.));
#1896=DIRECTION('center_axis',(0.,1.,0.));
#1897=DIRECTION('ref_axis',(0.,0.,1.));
#1898=DIRECTION('',(0.,1.,0.));
#1899=DIRECTION('center_axis',(0.,1.,0.));
#1900=DIRECTION('ref_axis',(0.,0.,1.));
#1901=DIRECTION('center_axis',(0.,1.,0.));
#1902=DIRECTION('ref_axis',(0.,0.,1.));
#1903=DIRECTION('center_axis',(0.,-1.,0.));
#1904=DIRECTION('ref_axis',(0.,0.,1.));
#1905=DIRECTION('',(0.,1.,0.));
#1906=DIRECTION('center_axis',(0.,-1.,0.));
#1907=DIRECTION('ref_axis',(0.,0.,1.));
#1908=DIRECTION('center_axis',(0.,1.,0.));
#1909=DIRECTION('ref_axis',(0.,0.,1.));
#1910=DIRECTION('center_axis',(0.,1.,0.));
#1911=DIRECTION('ref_axis',(0.,0.,1.));
#1912=DIRECTION('',(0.,1.,0.));
#1913=DIRECTION('center_axis',(0.,1.,0.));
#1914=DIRECTION('ref_axis',(0.,0.,1.));
#1915=DIRECTION('center_axis',(0.,1.,0.));
#1916=DIRECTION('ref_axis',(0.,0.,1.));
#1917=DIRECTION('',(1.,0.,0.));
#1918=DIRECTION('',(0.,0.,-1.));
#1919=DIRECTION('',(1.,0.,0.));
#1920=DIRECTION('',(0.,0.,-1.));
#1921=DIRECTION('center_axis',(0.,1.,0.));
#1922=DIRECTION('ref_axis',(0.,0.,1.));
#1923=DIRECTION('',(1.,0.,0.));
#1924=DIRECTION('',(0.,0.,-1.));
#1925=DIRECTION('',(1.,0.,0.));
#1926=DIRECTION('',(0.,0.,-1.));
#1927=DIRECTION('center_axis',(0.,1.,0.));
#1928=DIRECTION('ref_axis',(0.,0.,1.));
#1929=DIRECTION('',(1.,0.,0.));
#1930=DIRECTION('',(0.,0.,-1.));
#1931=DIRECTION('',(-1.,0.,0.));
#1932=DIRECTION('',(0.,0.,-1.));
#1933=DIRECTION('',(-1.,0.,0.));
#1934=DIRECTION('',(0.,0.,1.));
#1935=DIRECTION('',(1.,0.,0.));
#1936=DIRECTION('',(0.,0.,-1.));
#1937=DIRECTION('center_axis',(0.,1.,0.));
#1938=DIRECTION('ref_axis',(0.,0.,1.));
#1939=DIRECTION('',(0.,0.,-1.));
#1940=DIRECTION('',(1.,0.,0.));
#1941=DIRECTION('',(0.,0.,-1.));
#1942=DIRECTION('',(1.,0.,0.));
#1943=DIRECTION('',(0.,0.,-1.));
#1944=DIRECTION('',(1.,0.,0.));
#1945=DIRECTION('',(0.,0.,1.));
#1946=DIRECTION('',(1.,0.,0.));
#1947=DIRECTION('center_axis',(0.,0.,-1.));
#1948=DIRECTION('ref_axis',(-1.,0.,0.));
#1949=DIRECTION('',(-1.,0.,0.));
#1950=DIRECTION('',(0.,1.,0.));
#1951=DIRECTION('',(0.,-1.,0.));
#1952=DIRECTION('',(0.,1.,0.));
#1953=DIRECTION('center_axis',(0.,0.,1.));
#1954=DIRECTION('ref_axis',(1.,0.,0.));
#1955=DIRECTION('',(-1.,0.,0.));
#1956=DIRECTION('',(0.,1.,0.));
#1957=DIRECTION('',(0.,-1.,0.));
#1958=DIRECTION('',(0.,-1.,0.));
#1959=DIRECTION('center_axis',(1.,0.,0.));
#1960=DIRECTION('ref_axis',(0.,0.,-1.));
#1961=DIRECTION('',(0.,1.,0.));
#1962=DIRECTION('',(0.,0.,-1.));
#1963=DIRECTION('',(0.,-1.,0.));
#1964=DIRECTION('',(0.,0.,1.));
#1965=DIRECTION('',(0.,1.,0.));
#1966=DIRECTION('center_axis',(-1.,0.,0.));
#1967=DIRECTION('ref_axis',(0.,0.,1.));
#1968=DIRECTION('',(0.,0.,1.));
#1969=DIRECTION('',(0.,1.,0.));
#1970=DIRECTION('',(0.,1.,0.));
#1971=DIRECTION('',(0.,0.,1.));
#1972=DIRECTION('',(0.,1.,0.));
#1973=DIRECTION('center_axis',(0.,0.,1.));
#1974=DIRECTION('ref_axis',(1.,0.,0.));
#1975=DIRECTION('',(-0.270221787772536,-0.962798102102935,0.));
#1976=DIRECTION('center_axis',(0.,0.,-1.));
#1977=DIRECTION('ref_axis',(1.,1.15648231731787E-14,0.));
#1978=DIRECTION('',(0.,1.,0.));
#1979=DIRECTION('center_axis',(0.,0.,-1.));
#1980=DIRECTION('ref_axis',(1.,5.72458747072346E-14,0.));
#1981=DIRECTION('center_axis',(0.,0.,1.));
#1982=DIRECTION('ref_axis',(1.,0.,0.));
#1983=DIRECTION('',(0.962798102102935,-0.270221787772537,0.));
#1984=DIRECTION('',(0.962798102102935,-0.270221787772537,0.));
#1985=DIRECTION('',(0.270221787772547,0.962798102102932,0.));
#1986=DIRECTION('center_axis',(0.,0.,-1.));
#1987=DIRECTION('ref_axis',(-1.,0.,0.));
#1988=DIRECTION('center_axis',(0.,0.,-1.));
#1989=DIRECTION('ref_axis',(1.,1.15648231731787E-14,0.));
#1990=DIRECTION('',(0.270221787772536,0.962798102102935,0.));
#1991=DIRECTION('center_axis',(0.,0.,-1.));
#1992=DIRECTION('ref_axis',(1.,5.72458747072346E-14,0.));
#1993=DIRECTION('center_axis',(0.,0.,1.));
#1994=DIRECTION('ref_axis',(1.,0.,0.));
#1995=DIRECTION('',(0.,-1.,0.));
#1996=DIRECTION('center_axis',(0.,0.,1.));
#1997=DIRECTION('ref_axis',(-1.,1.11022302462516E-13,0.));
#1998=DIRECTION('center_axis',(0.,0.,1.));
#1999=DIRECTION('ref_axis',(1.,0.,0.));
#2000=DIRECTION('center_axis',(0.,0.,1.));
#2001=DIRECTION('ref_axis',(1.,0.,0.));
#2002=DIRECTION('',(1.,0.,0.));
#2003=DIRECTION('',(1.,0.,0.));
#2004=DIRECTION('',(0.,1.,0.));
#2005=DIRECTION('center_axis',(0.,0.,-1.));
#2006=DIRECTION('ref_axis',(-1.,0.,0.));
#2007=DIRECTION('',(-0.270221787772547,-0.962798102102932,0.));
#2008=DIRECTION('center_axis',(0.,0.,1.));
#2009=DIRECTION('ref_axis',(-1.,1.11022302462516E-13,0.));
#2010=DIRECTION('',(0.,1.,0.));
#2011=DIRECTION('center_axis',(0.,0.,1.));
#2012=DIRECTION('ref_axis',(1.,0.,0.));
#2013=DIRECTION('center_axis',(0.,0.,-1.));
#2014=DIRECTION('ref_axis',(-1.,0.,0.));
#2015=DIRECTION('',(0.962798102102935,-0.270221787772537,0.));
#2016=DIRECTION('',(0.962798102102935,-0.270221787772537,0.));
#2017=DIRECTION('center_axis',(0.,0.,1.));
#2018=DIRECTION('ref_axis',(1.,0.,0.));
#2019=DIRECTION('',(0.27022178777254,-0.962798102102934,0.));
#2020=DIRECTION('center_axis',(0.,0.,1.));
#2021=DIRECTION('ref_axis',(-1.,2.08166817117217E-14,0.));
#2022=DIRECTION('center_axis',(0.,0.,1.));
#2023=DIRECTION('ref_axis',(1.,0.,0.));
#2024=DIRECTION('center_axis',(0.,0.,1.));
#2025=DIRECTION('ref_axis',(1.,0.,0.));
#2026=DIRECTION('',(0.962798102102935,0.270221787772537,0.));
#2027=DIRECTION('',(0.962798102102935,0.270221787772537,0.));
#2028=DIRECTION('',(-0.270221787772533,0.962798102102936,0.));
#2029=DIRECTION('center_axis',(0.,0.,-1.));
#2030=DIRECTION('ref_axis',(-1.,0.,0.));
#2031=DIRECTION('',(0.,-1.,0.));
#2032=DIRECTION('center_axis',(0.,0.,1.));
#2033=DIRECTION('ref_axis',(-1.,2.08166817117217E-14,0.));
#2034=DIRECTION('',(-0.27022178777254,0.962798102102934,0.));
#2035=DIRECTION('center_axis',(0.,0.,1.));
#2036=DIRECTION('ref_axis',(1.,0.,0.));
#2037=DIRECTION('center_axis',(0.,0.,-1.));
#2038=DIRECTION('ref_axis',(-1.,0.,0.));
#2039=DIRECTION('',(1.,0.,0.));
#2040=DIRECTION('',(1.,0.,0.));
#2041=DIRECTION('center_axis',(0.,0.,1.));
#2042=DIRECTION('ref_axis',(1.,0.,0.));
#2043=DIRECTION('center_axis',(0.,0.,-1.));
#2044=DIRECTION('ref_axis',(1.,4.48431918959993E-15,0.));
#2045=DIRECTION('center_axis',(0.,0.,-1.));
#2046=DIRECTION('ref_axis',(1.,-1.12757025938492E-14,0.));
#2047=DIRECTION('center_axis',(0.,0.,-1.));
#2048=DIRECTION('ref_axis',(-1.,0.,0.));
#2049=DIRECTION('',(0.270221787772533,-0.962798102102936,0.));
#2050=DIRECTION('center_axis',(0.,0.,-1.));
#2051=DIRECTION('ref_axis',(1.,4.48431918959993E-15,0.));
#2052=DIRECTION('',(0.,1.,0.));
#2053=DIRECTION('center_axis',(0.,0.,-1.));
#2054=DIRECTION('ref_axis',(1.,-1.12757025938492E-14,0.));
#2055=DIRECTION('center_axis',(0.,0.,-1.));
#2056=DIRECTION('ref_axis',(-1.,0.,0.));
#2057=DIRECTION('',(0.962798102102935,0.270221787772537,0.));
#2058=DIRECTION('',(0.962798102102935,0.270221787772537,0.));
#2059=DIRECTION('center_axis',(0.,0.,-1.));
#2060=DIRECTION('ref_axis',(-1.,0.,0.));
#2061=DIRECTION('',(0.,0.,-1.));
#2062=DIRECTION('center_axis',(-0.270221787772537,0.962798102102935,0.));
#2063=DIRECTION('ref_axis',(-0.962798102102935,-0.270221787772537,0.));
#2064=DIRECTION('',(0.,0.,-1.));
#2065=DIRECTION('center_axis',(0.,0.,-1.));
#2066=DIRECTION('ref_axis',(-1.,0.,0.));
#2067=DIRECTION('',(0.,0.,-1.));
#2068=DIRECTION('center_axis',(0.,1.,0.));
#2069=DIRECTION('ref_axis',(0.,0.,1.));
#2070=DIRECTION('',(0.,0.,-1.));
#2071=DIRECTION('center_axis',(0.,0.,-1.));
#2072=DIRECTION('ref_axis',(-1.,0.,0.));
#2073=DIRECTION('',(0.,0.,-1.));
#2074=DIRECTION('center_axis',(0.270221787772537,0.962798102102935,0.));
#2075=DIRECTION('ref_axis',(-0.962798102102935,0.270221787772537,0.));
#2076=DIRECTION('',(0.,0.,-1.));
#2077=DIRECTION('center_axis',(0.,0.,-1.));
#2078=DIRECTION('ref_axis',(-1.,0.,0.));
#2079=DIRECTION('center_axis',(0.,0.,-1.));
#2080=DIRECTION('ref_axis',(-1.,0.,0.));
#2081=DIRECTION('',(0.,0.,-1.));
#2082=DIRECTION('center_axis',(0.270221787772537,0.962798102102935,0.));
#2083=DIRECTION('ref_axis',(-0.962798102102935,0.270221787772537,0.));
#2084=DIRECTION('',(0.,0.,-1.));
#2085=DIRECTION('center_axis',(0.,0.,-1.));
#2086=DIRECTION('ref_axis',(-1.,0.,0.));
#2087=DIRECTION('',(0.,0.,-1.));
#2088=DIRECTION('center_axis',(0.,1.,0.));
#2089=DIRECTION('ref_axis',(0.,0.,1.));
#2090=DIRECTION('',(0.,0.,-1.));
#2091=DIRECTION('center_axis',(0.,0.,-1.));
#2092=DIRECTION('ref_axis',(-1.,0.,0.));
#2093=DIRECTION('',(0.,0.,-1.));
#2094=DIRECTION('center_axis',(-0.270221787772537,0.962798102102935,0.));
#2095=DIRECTION('ref_axis',(-0.962798102102935,-0.270221787772537,0.));
#2096=DIRECTION('',(0.,0.,-1.));
#2097=DIRECTION('center_axis',(0.,0.,-1.));
#2098=DIRECTION('ref_axis',(-1.,0.,0.));
#2099=DIRECTION('center_axis',(0.,0.,1.));
#2100=DIRECTION('ref_axis',(1.,0.,0.));
#2101=DIRECTION('',(0.,1.,0.));
#2102=DIRECTION('',(1.,0.,0.));
#2103=DIRECTION('center_axis',(0.,0.,1.));
#2104=DIRECTION('ref_axis',(1.,0.,0.));
#2105=DIRECTION('',(0.,1.,0.));
#2106=DIRECTION('',(-1.,0.,0.));
#2107=DIRECTION('center_axis',(0.,0.,-1.));
#2108=DIRECTION('ref_axis',(-1.,0.,0.));
#2109=DIRECTION('',(-1.,0.,0.));
#2110=DIRECTION('',(0.,1.,0.));
#2111=DIRECTION('center_axis',(-1.,0.,0.));
#2112=DIRECTION('ref_axis',(0.,0.,1.));
#2113=DIRECTION('',(0.,0.,1.));
#2114=DIRECTION('center_axis',(0.,1.,0.));
#2115=DIRECTION('ref_axis',(0.,0.,1.));
#2116=DIRECTION('center_axis',(0.,0.,1.));
#2117=DIRECTION('ref_axis',(1.,0.,0.));
#2118=DIRECTION('',(1.,0.,0.));
#2119=DIRECTION('',(0.,1.,0.));
#2120=DIRECTION('center_axis',(1.,0.,0.));
#2121=DIRECTION('ref_axis',(0.,0.,-1.));
#2122=DIRECTION('',(0.,0.,-1.));
#2123=DIRECTION('center_axis',(0.,1.,0.));
#2124=DIRECTION('ref_axis',(0.,0.,1.));
#2125=DIRECTION('center_axis',(-1.,0.,0.));
#2126=DIRECTION('ref_axis',(0.,0.,1.));
#2127=DIRECTION('',(0.,0.,1.));
#2128=DIRECTION('',(0.,1.,0.));
#2129=DIRECTION('center_axis',(0.,0.,1.));
#2130=DIRECTION('ref_axis',(1.,0.,0.));
#2131=DIRECTION('',(1.,0.,0.));
#2132=DIRECTION('center_axis',(0.,1.,0.));
#2133=DIRECTION('ref_axis',(0.,0.,1.));
#2134=DIRECTION('center_axis',(1.,0.,0.));
#2135=DIRECTION('ref_axis',(0.,0.,-1.));
#2136=DIRECTION('',(0.,0.,-1.));
#2137=DIRECTION('',(0.,1.,0.));
#2138=DIRECTION('center_axis',(0.,0.,-1.));
#2139=DIRECTION('ref_axis',(-1.,0.,0.));
#2140=DIRECTION('',(-1.,0.,0.));
#2141=DIRECTION('center_axis',(0.,1.,0.));
#2142=DIRECTION('ref_axis',(0.,0.,1.));
#2331=CARTESIAN_POINT('',(0.,0.,0.));
#2332=CARTESIAN_POINT('Origin',(575.,7.00000000000001,12.7000000000002));
#2333=CARTESIAN_POINT('',(575.,-3.,19.7000000000001));
#2334=CARTESIAN_POINT('Origin',(575.,-3.,12.7000000000002));
#2335=CARTESIAN_POINT('',(575.,-6.34999999999999,19.7000000000001));
#2336=CARTESIAN_POINT('',(575.,7.00000000000001,19.7000000000001));
#2337=CARTESIAN_POINT('Origin',(575.,-6.34999999999999,12.7000000000002));
#2338=CARTESIAN_POINT('Origin',(25.,7.00000000000001,974.6));
#2339=CARTESIAN_POINT('',(25.,-3.,981.6));
#2340=CARTESIAN_POINT('Origin',(25.,-3.,974.6));
#2341=CARTESIAN_POINT('',(25.,-6.34999999999999,981.6));
#2342=CARTESIAN_POINT('',(25.,7.00000000000001,981.6));
#2343=CARTESIAN_POINT('Origin',(25.,-6.34999999999999,974.6));
#2344=CARTESIAN_POINT('Origin',(25.,7.00000000000001,12.7000000000002));
#2345=CARTESIAN_POINT('',(25.,-3.,19.7000000000001));
#2346=CARTESIAN_POINT('Origin',(25.,-3.,12.7000000000002));
#2347=CARTESIAN_POINT('',(25.,-6.34999999999999,19.7000000000001));
#2348=CARTESIAN_POINT('',(25.,7.00000000000001,19.7000000000001));
#2349=CARTESIAN_POINT('Origin',(25.,-6.34999999999999,12.7000000000002));
#2350=CARTESIAN_POINT('Origin',(575.,7.00000000000001,974.6));
#2351=CARTESIAN_POINT('',(575.,-3.,981.6));
#2352=CARTESIAN_POINT('Origin',(575.,-3.,974.6));
#2353=CARTESIAN_POINT('',(575.,-6.34999999999999,981.6));
#2354=CARTESIAN_POINT('',(575.,7.00000000000001,981.6));
#2355=CARTESIAN_POINT('Origin',(575.,-6.34999999999999,974.6));
#2356=CARTESIAN_POINT('Origin',(562.5,-10.,50.));
#2357=CARTESIAN_POINT('',(562.5,-6.34999999999999,28.5));
#2358=CARTESIAN_POINT('Origin',(562.5,-6.34999999999999,50.));
#2359=CARTESIAN_POINT('',(562.5,0.,28.5));
#2360=CARTESIAN_POINT('',(562.5,-10.,28.5));
#2361=CARTESIAN_POINT('Origin',(562.5,0.,50.));
#2362=CARTESIAN_POINT('Origin',(562.5,-10.,937.3));
#2363=CARTESIAN_POINT('',(562.5,-6.34999999999999,915.8));
#2364=CARTESIAN_POINT('Origin',(562.5,-6.34999999999999,937.3));
#2365=CARTESIAN_POINT('',(562.5,0.,915.8));
#2366=CARTESIAN_POINT('',(562.5,-10.,915.8));
#2367=CARTESIAN_POINT('Origin',(562.5,0.,937.3));
#2368=CARTESIAN_POINT('Origin',(37.4999999999998,-10.,937.3));
#2369=CARTESIAN_POINT('',(37.4999999999998,-6.34999999999999,915.8));
#2370=CARTESIAN_POINT('Origin',(37.4999999999998,-6.34999999999999,937.3));
#2371=CARTESIAN_POINT('',(37.4999999999998,0.,915.8));
#2372=CARTESIAN_POINT('',(37.4999999999998,-10.,915.8));
#2373=CARTESIAN_POINT('Origin',(37.4999999999998,0.,937.3));
#2374=CARTESIAN_POINT('Origin',(37.4999999999998,-10.,50.));
#2375=CARTESIAN_POINT('',(37.4999999999998,-6.34999999999999,28.5));
#2376=CARTESIAN_POINT('Origin',(37.4999999999998,-6.34999999999999,50.));
#2377=CARTESIAN_POINT('',(37.4999999999998,0.,28.5));
#2378=CARTESIAN_POINT('',(37.4999999999998,-10.,28.5));
#2379=CARTESIAN_POINT('Origin',(37.4999999999998,0.,50.));
#2380=CARTESIAN_POINT('Origin',(520.,-6.34999999999999,987.3));
#2381=CARTESIAN_POINT('',(521.011887130928,-6.34999999999999,0.));
#2382=CARTESIAN_POINT('',(600.,-6.34999999999999,0.));
#2383=CARTESIAN_POINT('',(520.,-6.34999999999999,0.));
#2384=CARTESIAN_POINT('',(600.,-6.34999999999999,987.3));
#2385=CARTESIAN_POINT('',(600.,-6.34999999999999,987.3));
#2386=CARTESIAN_POINT('',(521.011887130928,-6.34999999999999,987.3));
#2387=CARTESIAN_POINT('',(520.,-6.34999999999999,987.3));
#2388=CARTESIAN_POINT('',(521.011887130928,-6.34999999999999,987.3));
#2389=CARTESIAN_POINT('Origin',(0.,-6.34999999999999,987.3));
#2390=CARTESIAN_POINT('',(0.,-6.34999999999999,0.));
#2391=CARTESIAN_POINT('',(78.9881128690719,-6.34999999999999,0.));
#2392=CARTESIAN_POINT('',(0.,-6.34999999999999,0.));
#2393=CARTESIAN_POINT('',(78.9881128690719,-6.34999999999999,987.3));
#2394=CARTESIAN_POINT('',(78.9881128690719,-6.34999999999999,987.3));
#2395=CARTESIAN_POINT('',(0.,-6.34999999999999,987.3));
#2396=CARTESIAN_POINT('',(0.,-6.34999999999999,987.3));
#2397=CARTESIAN_POINT('',(0.,-6.34999999999999,987.3));
#2398=CARTESIAN_POINT('Origin',(520.,0.,987.3));
#2399=CARTESIAN_POINT('',(521.011887130928,0.,987.3));
#2400=CARTESIAN_POINT('',(555.,0.,987.3));
#2401=CARTESIAN_POINT('',(520.,0.,987.3));
#2402=CARTESIAN_POINT('',(555.,0.,962.3));
#2403=CARTESIAN_POINT('',(555.,0.,0.));
#2404=CARTESIAN_POINT('',(600.,0.,962.3));
#2405=CARTESIAN_POINT('',(0.,0.,962.3));
#2406=CARTESIAN_POINT('',(600.,0.,25.));
#2407=CARTESIAN_POINT('',(600.,0.,987.3));
#2408=CARTESIAN_POINT('',(555.,0.,25.));
#2409=CARTESIAN_POINT('',(0.,0.,25.));
#2410=CARTESIAN_POINT('',(555.,0.,0.));
#2411=CARTESIAN_POINT('',(555.,0.,0.));
#2412=CARTESIAN_POINT('',(521.011887130928,0.,0.));
#2413=CARTESIAN_POINT('',(520.,0.,0.));
#2414=CARTESIAN_POINT('',(521.011887130928,0.,987.3));
#2415=CARTESIAN_POINT('Origin',(0.,0.,987.3));
#2416=CARTESIAN_POINT('',(0.,0.,962.3));
#2417=CARTESIAN_POINT('',(0.,0.,25.));
#2418=CARTESIAN_POINT('',(0.,0.,987.3));
#2419=CARTESIAN_POINT('',(45.,0.,962.3));
#2420=CARTESIAN_POINT('',(0.,0.,962.3));
#2421=CARTESIAN_POINT('',(45.,0.,987.3));
#2422=CARTESIAN_POINT('',(45.,0.,0.));
#2423=CARTESIAN_POINT('',(78.9881128690719,0.,987.3));
#2424=CARTESIAN_POINT('',(0.,0.,987.3));
#2425=CARTESIAN_POINT('',(78.9881128690719,0.,0.));
#2426=CARTESIAN_POINT('',(78.9881128690719,0.,987.3));
#2427=CARTESIAN_POINT('',(44.9999999999999,0.,0.));
#2428=CARTESIAN_POINT('',(0.,0.,0.));
#2429=CARTESIAN_POINT('',(44.9999999999999,0.,25.));
#2430=CARTESIAN_POINT('',(44.9999999999999,0.,0.));
#2431=CARTESIAN_POINT('',(0.,0.,25.));
#2432=CARTESIAN_POINT('Origin',(79.2583346568445,-6.38720189789707,0.));
#2433=CARTESIAN_POINT('',(44.9999999999999,-3.,0.));
#2434=CARTESIAN_POINT('',(0.,-3.,0.));
#2435=CARTESIAN_POINT('',(0.,-3.,0.));
#2436=CARTESIAN_POINT('',(44.9999999999999,-3.,0.));
#2437=CARTESIAN_POINT('',(78.9881128690719,0.,0.));
#2438=CARTESIAN_POINT('',(0.,-6.34999999999999,0.));
#2439=CARTESIAN_POINT('Origin',(520.741665343155,-6.3872018978971,987.3));
#2440=CARTESIAN_POINT('',(600.,-3.,987.3));
#2441=CARTESIAN_POINT('',(555.,-3.,987.3));
#2442=CARTESIAN_POINT('',(0.,-3.,987.3));
#2443=CARTESIAN_POINT('',(555.,-3.,987.3));
#2444=CARTESIAN_POINT('',(521.011887130928,0.,987.3));
#2445=CARTESIAN_POINT('',(600.,0.,987.3));
#2446=CARTESIAN_POINT('Origin',(600.,0.,987.3));
#2447=CARTESIAN_POINT('',(600.,-3.,962.3));
#2448=CARTESIAN_POINT('',(600.,-3.,962.3));
#2449=CARTESIAN_POINT('',(600.,-3.,0.));
#2450=CARTESIAN_POINT('',(600.,-3.,0.));
#2451=CARTESIAN_POINT('',(600.,0.,0.));
#2452=CARTESIAN_POINT('',(600.,-3.,25.));
#2453=CARTESIAN_POINT('',(600.,-3.,0.));
#2454=CARTESIAN_POINT('',(600.,-3.,25.));
#2455=CARTESIAN_POINT('Origin',(0.,-6.34999999999999,987.3));
#2456=CARTESIAN_POINT('',(0.,-3.,962.3));
#2457=CARTESIAN_POINT('',(0.,-3.,987.3));
#2458=CARTESIAN_POINT('',(0.,-3.,0.));
#2459=CARTESIAN_POINT('',(0.,-3.,962.3));
#2460=CARTESIAN_POINT('',(0.,-3.,25.));
#2461=CARTESIAN_POINT('',(0.,-3.,25.));
#2462=CARTESIAN_POINT('',(0.,-3.,0.));
#2463=CARTESIAN_POINT('',(0.,-6.34999999999999,987.3));
#2464=CARTESIAN_POINT('Origin',(80.9742430092,-0.273433949543433,987.3));
#2465=CARTESIAN_POINT('',(80.9742430092,-0.273433949543433,987.3));
#2466=CARTESIAN_POINT('',(79.2583346568445,-6.38720189789707,987.3));
#2467=CARTESIAN_POINT('',(80.9742430092,-0.273433949543433,987.3));
#2468=CARTESIAN_POINT('Origin',(78.9881128690719,-7.35,987.3));
#2469=CARTESIAN_POINT('',(78.9881128690719,-6.34999999999999,987.3));
#2470=CARTESIAN_POINT('Origin',(78.9881128690719,-7.35,987.3));
#2471=CARTESIAN_POINT('Origin',(78.9881128690719,-6.34999999999999,987.3));
#2472=CARTESIAN_POINT('',(260.867449930721,-50.7627981021028,987.3));
#2473=CARTESIAN_POINT('',(80.,0.,987.3));
#2474=CARTESIAN_POINT('',(259.151541578365,-56.8765660504565,987.3));
#2475=CARTESIAN_POINT('',(78.2840916476444,-6.11376794835364,987.3));
#2476=CARTESIAN_POINT('',(259.151541578365,-56.8765660504565,987.3));
#2477=CARTESIAN_POINT('Origin',(78.9881128690719,0.,0.));
#2478=CARTESIAN_POINT('',(80.9742430092,-0.273433949543433,0.));
#2479=CARTESIAN_POINT('Origin',(78.9881128690719,-7.35,0.));
#2480=CARTESIAN_POINT('',(79.2583346568445,-6.38720189789707,0.));
#2481=CARTESIAN_POINT('',(79.2583346568445,-6.38720189789707,0.));
#2482=CARTESIAN_POINT('Origin',(78.9881128690719,-7.35,0.));
#2483=CARTESIAN_POINT('Origin',(261.137671718493,-50.8,987.3));
#2484=CARTESIAN_POINT('',(261.137671718493,-50.8,987.3));
#2485=CARTESIAN_POINT('',(261.137671718493,-57.15,987.3));
#2486=CARTESIAN_POINT('',(261.137671718493,-50.8,987.3));
#2487=CARTESIAN_POINT('Origin',(261.137671718493,-49.8,987.3));
#2488=CARTESIAN_POINT('Origin',(261.137671718493,-49.8,987.3));
#2489=CARTESIAN_POINT('Origin',(259.151541578365,-56.8765660504565,987.3));
#2490=CARTESIAN_POINT('',(338.862328281506,-50.8,987.3));
#2491=CARTESIAN_POINT('',(261.,-50.8,987.3));
#2492=CARTESIAN_POINT('',(338.862328281506,-57.15,987.3));
#2493=CARTESIAN_POINT('',(261.,-57.15,987.3));
#2494=CARTESIAN_POINT('',(338.862328281506,-57.15,987.3));
#2495=CARTESIAN_POINT('Origin',(260.867449930721,-50.7627981021028,0.));
#2496=CARTESIAN_POINT('',(260.867449930721,-50.7627981021028,0.));
#2497=CARTESIAN_POINT('',(259.151541578365,-56.8765660504565,0.));
#2498=CARTESIAN_POINT('',(260.867449930721,-50.7627981021028,0.));
#2499=CARTESIAN_POINT('',(261.137671718493,-50.8,0.));
#2500=CARTESIAN_POINT('Origin',(261.137671718493,-49.8,0.));
#2501=CARTESIAN_POINT('',(261.137671718493,-57.15,0.));
#2502=CARTESIAN_POINT('',(261.137671718493,-57.15,0.));
#2503=CARTESIAN_POINT('Origin',(261.137671718493,-49.8,0.));
#2504=CARTESIAN_POINT('Origin',(261.137671718493,-57.15,0.));
#2505=CARTESIAN_POINT('',(80.,0.,0.));
#2506=CARTESIAN_POINT('',(78.2840916476444,-6.11376794835364,0.));
#2507=CARTESIAN_POINT('Origin',(339.132550069279,-50.7627981021029,987.3));
#2508=CARTESIAN_POINT('',(339.132550069279,-50.7627981021029,987.3));
#2509=CARTESIAN_POINT('',(340.848458421635,-56.8765660504566,987.3));
#2510=CARTESIAN_POINT('',(339.132550069279,-50.7627981021029,987.3));
#2511=CARTESIAN_POINT('Origin',(338.862328281506,-49.8,987.3));
#2512=CARTESIAN_POINT('Origin',(338.862328281506,-49.8,987.3));
#2513=CARTESIAN_POINT('Origin',(338.862328281506,-57.15,987.3));
#2514=CARTESIAN_POINT('',(519.0257569908,-0.273433949543461,987.3));
#2515=CARTESIAN_POINT('',(339.,-50.8,987.3));
#2516=CARTESIAN_POINT('',(520.741665343155,-6.3872018978971,987.3));
#2517=CARTESIAN_POINT('',(340.715908352356,-56.9137679483536,987.3));
#2518=CARTESIAN_POINT('',(520.741665343155,-6.3872018978971,987.3));
#2519=CARTESIAN_POINT('Origin',(338.862328281506,-50.8,0.));
#2520=CARTESIAN_POINT('',(338.862328281506,-50.8,0.));
#2521=CARTESIAN_POINT('',(338.862328281506,-57.15,0.));
#2522=CARTESIAN_POINT('',(338.862328281506,-50.8,0.));
#2523=CARTESIAN_POINT('',(339.132550069279,-50.7627981021029,0.));
#2524=CARTESIAN_POINT('Origin',(338.862328281506,-49.8,0.));
#2525=CARTESIAN_POINT('',(340.848458421635,-56.8765660504566,0.));
#2526=CARTESIAN_POINT('',(340.848458421635,-56.8765660504566,0.));
#2527=CARTESIAN_POINT('Origin',(338.862328281506,-49.8,0.));
#2528=CARTESIAN_POINT('Origin',(340.848458421635,-56.8765660504566,0.));
#2529=CARTESIAN_POINT('',(261.,-50.8,0.));
#2530=CARTESIAN_POINT('',(261.,-57.15,0.));
#2531=CARTESIAN_POINT('Origin',(521.011887130928,0.,987.3));
#2532=CARTESIAN_POINT('Origin',(521.011887130928,-7.35000000000002,987.3));
#2533=CARTESIAN_POINT('Origin',(521.011887130928,-7.35000000000002,987.3));
#2534=CARTESIAN_POINT('Origin',(519.0257569908,-0.273433949543461,0.));
#2535=CARTESIAN_POINT('',(519.0257569908,-0.273433949543461,0.));
#2536=CARTESIAN_POINT('',(520.741665343155,-6.3872018978971,0.));
#2537=CARTESIAN_POINT('',(519.0257569908,-0.273433949543461,0.));
#2538=CARTESIAN_POINT('Origin',(521.011887130928,-7.35000000000002,0.));
#2539=CARTESIAN_POINT('',(521.011887130928,-6.34999999999999,0.));
#2540=CARTESIAN_POINT('Origin',(521.011887130928,-7.35000000000002,0.));
#2541=CARTESIAN_POINT('Origin',(521.011887130928,-6.34999999999999,0.));
#2542=CARTESIAN_POINT('',(339.,-50.8,0.));
#2543=CARTESIAN_POINT('',(340.715908352356,-56.9137679483536,0.));
#2544=CARTESIAN_POINT('Origin',(521.011887130928,-7.35000000000002,987.3));
#2545=CARTESIAN_POINT('',(519.0257569908,-0.273433949543461,987.3));
#2546=CARTESIAN_POINT('Origin',(339.,-50.8,987.3));
#2547=CARTESIAN_POINT('',(339.132550069279,-50.7627981021029,987.3));
#2548=CARTESIAN_POINT('Origin',(338.862328281506,-49.8,987.3));
#2549=CARTESIAN_POINT('',(338.862328281506,-50.8,987.3));
#2550=CARTESIAN_POINT('Origin',(261.,-50.8,987.3));
#2551=CARTESIAN_POINT('',(261.137671718493,-50.8,987.3));
#2552=CARTESIAN_POINT('Origin',(261.137671718493,-49.8,987.3));
#2553=CARTESIAN_POINT('',(260.867449930721,-50.7627981021028,987.3));
#2554=CARTESIAN_POINT('Origin',(80.,0.,987.3));
#2555=CARTESIAN_POINT('',(80.9742430092,-0.273433949543433,987.3));
#2556=CARTESIAN_POINT('Origin',(78.9881128690719,-7.35,987.3));
#2557=CARTESIAN_POINT('Origin',(78.9881128690719,-7.35,987.3));
#2558=CARTESIAN_POINT('',(79.2583346568445,-6.38720189789707,987.3));
#2559=CARTESIAN_POINT('Origin',(78.2840916476444,-6.11376794835364,987.3));
#2560=CARTESIAN_POINT('',(259.151541578365,-56.8765660504565,987.3));
#2561=CARTESIAN_POINT('Origin',(261.137671718493,-49.8,987.3));
#2562=CARTESIAN_POINT('',(261.137671718493,-57.15,987.3));
#2563=CARTESIAN_POINT('Origin',(261.,-57.15,987.3));
#2564=CARTESIAN_POINT('',(338.862328281506,-57.15,987.3));
#2565=CARTESIAN_POINT('Origin',(338.862328281506,-49.8,987.3));
#2566=CARTESIAN_POINT('',(340.848458421635,-56.8765660504566,987.3));
#2567=CARTESIAN_POINT('Origin',(340.715908352356,-56.9137679483536,987.3));
#2568=CARTESIAN_POINT('',(520.741665343155,-6.3872018978971,987.3));
#2569=CARTESIAN_POINT('Origin',(521.011887130928,-7.35000000000002,987.3));
#2570=CARTESIAN_POINT('Origin',(521.011887130928,-7.35000000000002,987.3));
#2571=CARTESIAN_POINT('',(45.,-3.,987.3));
#2572=CARTESIAN_POINT('',(45.,-3.,987.3));
#2573=CARTESIAN_POINT('',(0.,-3.,987.3));
#2574=CARTESIAN_POINT('Origin',(521.011887130928,-7.35000000000002,0.));
#2575=CARTESIAN_POINT('',(555.,-3.,0.));
#2576=CARTESIAN_POINT('',(555.,-3.,0.));
#2577=CARTESIAN_POINT('',(0.,-3.,0.));
#2578=CARTESIAN_POINT('Origin',(0.,-3.,25.));
#2579=CARTESIAN_POINT('',(555.,-3.,25.));
#2580=CARTESIAN_POINT('',(0.,-3.,25.));
#2581=CARTESIAN_POINT('',(555.,-3.,25.));
#2582=CARTESIAN_POINT('Origin',(555.,-3.,0.));
#2583=CARTESIAN_POINT('',(555.,-3.,0.));
#2584=CARTESIAN_POINT('Origin',(0.,-3.,0.));
#2585=CARTESIAN_POINT('Origin',(0.,-3.,962.3));
#2586=CARTESIAN_POINT('',(45.,-3.,962.3));
#2587=CARTESIAN_POINT('',(0.,-3.,962.3));
#2588=CARTESIAN_POINT('',(45.,-3.,962.3));
#2589=CARTESIAN_POINT('Origin',(45.,-3.,0.));
#2590=CARTESIAN_POINT('',(45.,-3.,0.));
#2591=CARTESIAN_POINT('Origin',(0.,-3.,0.));
#2592=CARTESIAN_POINT('Origin',(44.9999999999999,-3.,0.));
#2593=CARTESIAN_POINT('',(44.9999999999999,-3.,25.));
#2594=CARTESIAN_POINT('',(44.9999999999999,-3.,0.));
#2595=CARTESIAN_POINT('',(44.9999999999999,-3.,25.));
#2596=CARTESIAN_POINT('Origin',(0.,-3.,25.));
#2597=CARTESIAN_POINT('',(0.,-3.,25.));
#2598=CARTESIAN_POINT('Origin',(0.,-3.,0.));
#2599=CARTESIAN_POINT('Origin',(555.,-3.,0.));
#2600=CARTESIAN_POINT('',(555.,-3.,962.3));
#2601=CARTESIAN_POINT('',(555.,-3.,0.));
#2602=CARTESIAN_POINT('',(555.,-3.,962.3));
#2603=CARTESIAN_POINT('Origin',(0.,-3.,962.3));
#2604=CARTESIAN_POINT('',(0.,-3.,962.3));
#2605=CARTESIAN_POINT('Origin',(0.,-3.,0.));
#2782=UNCERTAINTY_MEASURE_WITH_UNIT(LENGTH_MEASURE(0.01),#2795,
'DISTANCE_ACCURACY_VALUE',
'Maximum model space distance between geometric entities at asserted c
onnectivities');
#2787=UNCERTAINTY_MEASURE_WITH_UNIT(LENGTH_MEASURE(0.01),#2795,
'DISTANCE_ACCURACY_VALUE',
'Maximum model space distance between geometric entities at asserted c
onnectivities');
#2789=(
GEOMETRIC_REPRESENTATION_CONTEXT(3)
GLOBAL_UNCERTAINTY_ASSIGNED_CONTEXT((#2782))
GLOBAL_UNIT_ASSIGNED_CONTEXT((#2795,#2797,#2798))
REPRESENTATION_CONTEXT('','3D')
);
#2794=(
GEOMETRIC_REPRESENTATION_CONTEXT(3)
GLOBAL_UNCERTAINTY_ASSIGNED_CONTEXT((#2787))
GLOBAL_UNIT_ASSIGNED_CONTEXT((#2795,#2797,#2798))
REPRESENTATION_CONTEXT('','3D')
);
#2795=(
LENGTH_UNIT()
NAMED_UNIT(*)
SI_UNIT(.MILLI.,.METRE.)
);
#2797=(
NAMED_UNIT(*)
PLANE_ANGLE_UNIT()
SI_UNIT($,.RADIAN.)
);
#2798=(
NAMED_UNIT(*)
SI_UNIT($,.STERADIAN.)
SOLID_ANGLE_UNIT()
);
#2800=SHAPE_DEFINITION_REPRESENTATION(#2806,#2827);
#2806=PRODUCT_DEFINITION_SHAPE('',$,#2834);
#2827=SHAPE_REPRESENTATION('',(#1703),#2789);
#2832=PRODUCT_DEFINITION_CONTEXT('part definition',#2852,'design');
#2834=PRODUCT_DEFINITION('Drilled Plate','Drilled Plate',#2840,#2832);
#2840=PRODUCT_DEFINITION_FORMATION('',$,#2855);
#2852=APPLICATION_CONTEXT(
'Core Data for Automotive Mechanical Design Process');
#2853=PRODUCT_CONTEXT('part definition',#2852,'mechanical');
#2855=PRODUCT('Drilled Plate','Drilled Plate',$,(#2853));
#2861=PRESENTATION_STYLE_ASSIGNMENT((#2865));
#2865=SURFACE_STYLE_USAGE(.BOTH.,#2869);
#2869=SURFACE_SIDE_STYLE('',(#2873));
#2873=SURFACE_STYLE_FILL_AREA(#2877);
#2877=FILL_AREA_STYLE('Opaque(97,158,199)',(#2881));
#2881=FILL_AREA_STYLE_COLOUR('Opaque(97,158,199)',#2885);
#2885=COLOUR_RGB('Opaque(97,158,199)',0.380392156862745,0.619607843137255,
0.780392156862745);
ENDSEC;
END-ISO-10303-21;
